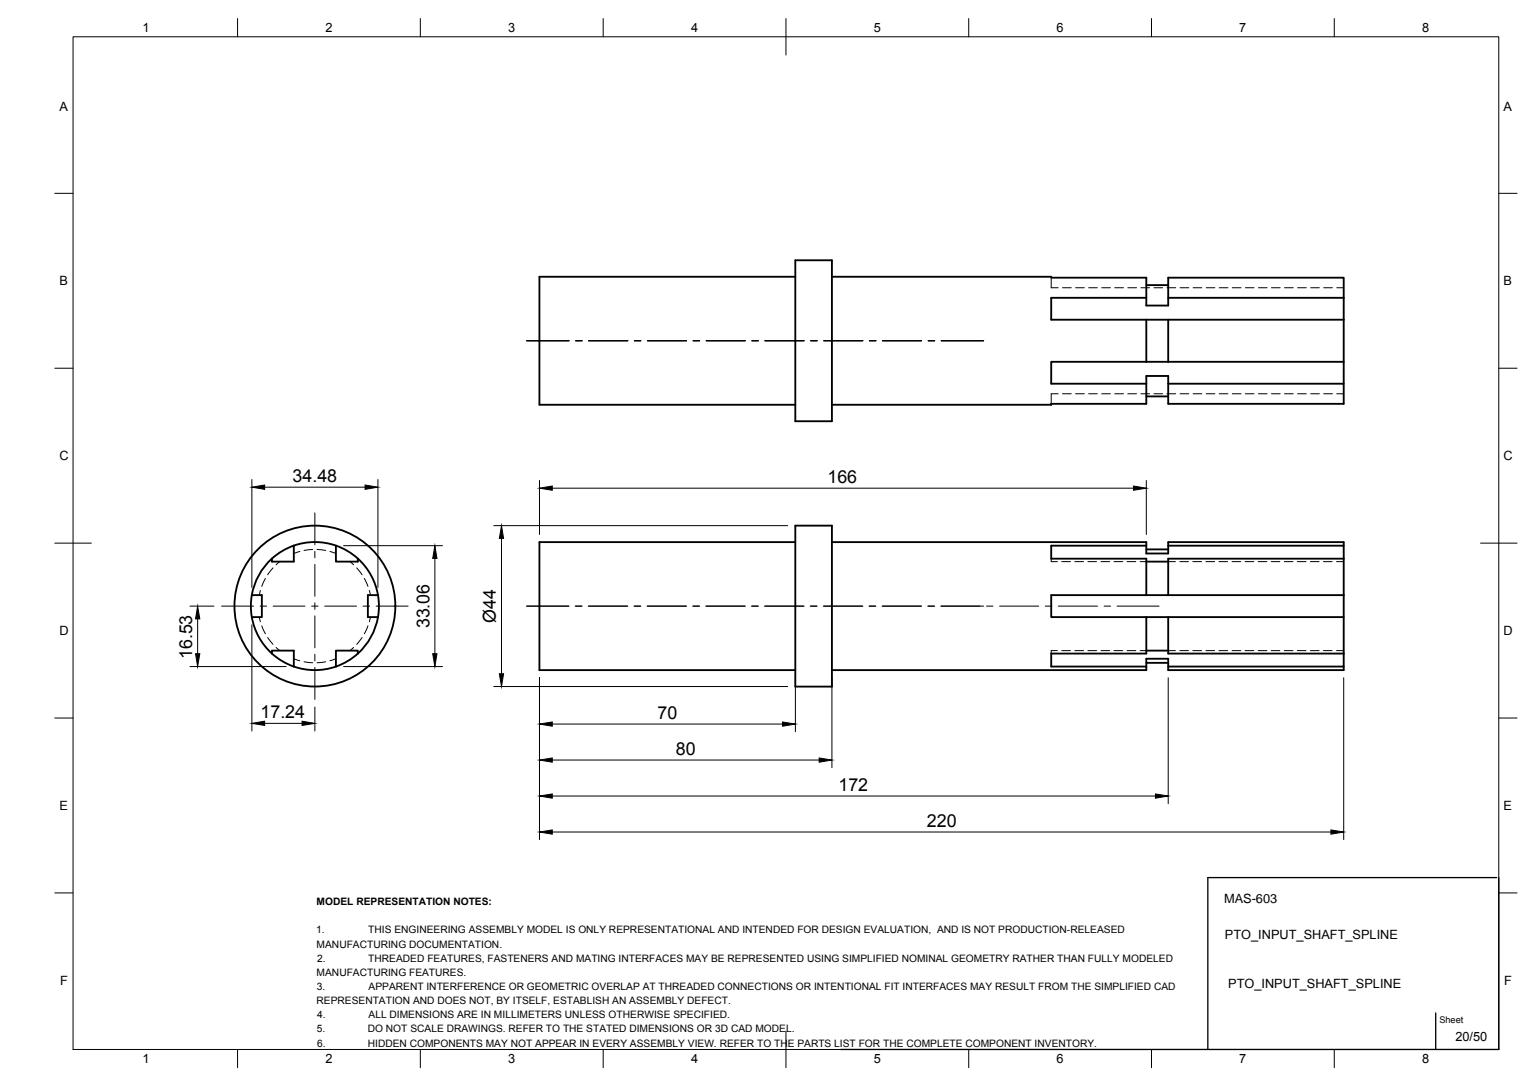
ISO-10303-21;
HEADER;
FILE_DESCRIPTION((''),'2;1');
FILE_NAME('PTO_INPUT_SHAFT_SPLINE.step','2026-10-01T22:06:14-07:00',(''),(''),'','','');
FILE_SCHEMA (('AUTOMOTIVE_DESIGN { 1 0 10303 214 3 1 1 }'));
ENDSEC;
DATA;
#10=MECHANICAL_DESIGN_GEOMETRIC_PRESENTATION_REPRESENTATION('',(#992),#50440);
#902=SHAPE_REPRESENTATION_RELATIONSHIP('SRR','None',#50634,#947) ;
#947=ADVANCED_BREP_SHAPE_REPRESENTATION('',(#1047),#50403) ;
#992=STYLED_ITEM('',(#50883),#1047) ;
#1047=MANIFOLD_SOLID_BREP('PTO_INPUT_SHAFT_SPLINE',#28659) ;
#1295=FACE_BOUND('',#4895,.T.) ;
#1296=FACE_BOUND('',#4898,.T.) ;
#1988=PLANE('',#30408) ;
#1989=PLANE('',#30411) ;
#1990=PLANE('',#30414) ;
#1991=PLANE('',#30417) ;
#1992=PLANE('',#30420) ;
#1993=PLANE('',#30423) ;
#1994=PLANE('',#30438) ;
#1995=PLANE('',#30440) ;
#1996=PLANE('',#30443) ;
#1997=PLANE('',#30445) ;
#1998=PLANE('',#30447) ;
#1999=PLANE('',#30449) ;
#2000=PLANE('',#30451) ;
#2001=PLANE('',#30452) ;
#2002=PLANE('',#30453) ;
#2003=PLANE('',#30454) ;
#2004=PLANE('',#30455) ;
#2005=PLANE('',#30456) ;
#2006=PLANE('',#30457) ;
#2007=PLANE('',#30458) ;
#2008=PLANE('',#30459) ;
#2009=PLANE('',#30460) ;
#2010=PLANE('',#30461) ;
#2011=PLANE('',#30462) ;
#2012=PLANE('',#30475) ;
#2013=PLANE('',#30477) ;
#2014=PLANE('',#30478) ;
#2015=PLANE('',#30479) ;
#2016=PLANE('',#30480) ;
#2017=PLANE('',#30481) ;
#2018=PLANE('',#30483) ;
#2019=PLANE('',#30485) ;
#2020=PLANE('',#30491) ;
#2021=PLANE('',#30492) ;
#2022=PLANE('',#30493) ;
#2023=PLANE('',#30494) ;
#2024=PLANE('',#30495) ;
#2025=PLANE('',#30496) ;
#2026=PLANE('',#30497) ;
#2027=PLANE('',#30498) ;
#2028=PLANE('',#30499) ;
#2029=PLANE('',#30503) ;
#2030=PLANE('',#30504) ;
#2031=PLANE('',#30508) ;
#3101=FACE_OUTER_BOUND('',#4838,.T.) ;
#3102=FACE_OUTER_BOUND('',#4839,.T.) ;
#3103=FACE_OUTER_BOUND('',#4840,.T.) ;
#3104=FACE_OUTER_BOUND('',#4841,.T.) ;
#3105=FACE_OUTER_BOUND('',#4842,.T.) ;
#3106=FACE_OUTER_BOUND('',#4843,.T.) ;
#3107=FACE_OUTER_BOUND('',#4844,.T.) ;
#3108=FACE_OUTER_BOUND('',#4845,.T.) ;
#3109=FACE_OUTER_BOUND('',#4846,.T.) ;
#3110=FACE_OUTER_BOUND('',#4847,.T.) ;
#3111=FACE_OUTER_BOUND('',#4848,.T.) ;
#3112=FACE_OUTER_BOUND('',#4849,.T.) ;
#3113=FACE_OUTER_BOUND('',#4850,.T.) ;
#3114=FACE_OUTER_BOUND('',#4851,.T.) ;
#3115=FACE_OUTER_BOUND('',#4852,.T.) ;
#3116=FACE_OUTER_BOUND('',#4853,.T.) ;
#3117=FACE_OUTER_BOUND('',#4854,.T.) ;
#3118=FACE_OUTER_BOUND('',#4855,.T.) ;
#3119=FACE_OUTER_BOUND('',#4856,.T.) ;
#3120=FACE_OUTER_BOUND('',#4857,.T.) ;
#3121=FACE_OUTER_BOUND('',#4858,.T.) ;
#3122=FACE_OUTER_BOUND('',#4859,.T.) ;
#3123=FACE_OUTER_BOUND('',#4860,.T.) ;
#3124=FACE_OUTER_BOUND('',#4861,.T.) ;
#3125=FACE_OUTER_BOUND('',#4862,.T.) ;
#3126=FACE_OUTER_BOUND('',#4863,.T.) ;
#3127=FACE_OUTER_BOUND('',#4864,.T.) ;
#3128=FACE_OUTER_BOUND('',#4865,.T.) ;
#3129=FACE_OUTER_BOUND('',#4866,.T.) ;
#3130=FACE_OUTER_BOUND('',#4867,.T.) ;
#3131=FACE_OUTER_BOUND('',#4868,.T.) ;
#3132=FACE_OUTER_BOUND('',#4869,.T.) ;
#3133=FACE_OUTER_BOUND('',#4870,.T.) ;
#3134=FACE_OUTER_BOUND('',#4871,.T.) ;
#3135=FACE_OUTER_BOUND('',#4872,.T.) ;
#3136=FACE_OUTER_BOUND('',#4873,.T.) ;
#3137=FACE_OUTER_BOUND('',#4874,.T.) ;
#3138=FACE_OUTER_BOUND('',#4875,.T.) ;
#3139=FACE_OUTER_BOUND('',#4876,.T.) ;
#3140=FACE_OUTER_BOUND('',#4877,.T.) ;
#3141=FACE_OUTER_BOUND('',#4878,.T.) ;
#3142=FACE_OUTER_BOUND('',#4879,.T.) ;
#3143=FACE_OUTER_BOUND('',#4880,.T.) ;
#3144=FACE_OUTER_BOUND('',#4881,.T.) ;
#3145=FACE_OUTER_BOUND('',#4882,.T.) ;
#3146=FACE_OUTER_BOUND('',#4883,.T.) ;
#3147=FACE_OUTER_BOUND('',#4884,.T.) ;
#3148=FACE_OUTER_BOUND('',#4885,.T.) ;
#3149=FACE_OUTER_BOUND('',#4886,.T.) ;
#3150=FACE_OUTER_BOUND('',#4887,.T.) ;
#3151=FACE_OUTER_BOUND('',#4888,.T.) ;
#3152=FACE_OUTER_BOUND('',#4889,.T.) ;
#3153=FACE_OUTER_BOUND('',#4890,.T.) ;
#3154=FACE_OUTER_BOUND('',#4891,.T.) ;
#3155=FACE_OUTER_BOUND('',#4892,.T.) ;
#3156=FACE_OUTER_BOUND('',#4893,.T.) ;
#3157=FACE_OUTER_BOUND('',#4894,.T.) ;
#3158=FACE_OUTER_BOUND('',#4896,.T.) ;
#3159=FACE_OUTER_BOUND('',#4897,.T.) ;
#4838=EDGE_LOOP('',(#22531,#22532,#22533,#22534,#22535)) ;
#4839=EDGE_LOOP('',(#22536,#22537,#22538,#22539,#22540)) ;
#4840=EDGE_LOOP('',(#22541,#22542,#22543,#22544)) ;
#4841=EDGE_LOOP('',(#22545,#22546,#22547,#22548,#22549)) ;
#4842=EDGE_LOOP('',(#22550,#22551,#22552,#22553,#22554)) ;
#4843=EDGE_LOOP('',(#22555,#22556,#22557,#22558)) ;
#4844=EDGE_LOOP('',(#22559,#22560,#22561,#22562)) ;
#4845=EDGE_LOOP('',(#22563,#22564,#22565,#22566)) ;
#4846=EDGE_LOOP('',(#22567,#22568,#22569,#22570)) ;
#4847=EDGE_LOOP('',(#22571,#22572,#22573,#22574)) ;
#4848=EDGE_LOOP('',(#22575,#22576,#22577,#22578)) ;
#4849=EDGE_LOOP('',(#22579,#22580,#22581,#22582)) ;
#4850=EDGE_LOOP('',(#22583,#22584,#22585,#22586,#22587)) ;
#4851=EDGE_LOOP('',(#22588,#22589,#22590,#22591,#22592)) ;
#4852=EDGE_LOOP('',(#22593,#22594,#22595,#22596,#22597)) ;
#4853=EDGE_LOOP('',(#22598,#22599,#22600,#22601,#22602)) ;
#4854=EDGE_LOOP('',(#22603,#22604,#22605,#22606,#22607)) ;
#4855=EDGE_LOOP('',(#22608,#22609,#22610,#22611)) ;
#4856=EDGE_LOOP('',(#22612,#22613,#22614,#22615,#22616,#22617,#22618,#22619)) ;
#4857=EDGE_LOOP('',(#22620,#22621,#22622,#22623,#22624,#22625,#22626,#22627)) ;
#4858=EDGE_LOOP('',(#22628,#22629,#22630,#22631)) ;
#4859=EDGE_LOOP('',(#22632,#22633,#22634,#22635,#22636,#22637,#22638,#22639)) ;
#4860=EDGE_LOOP('',(#22640,#22641,#22642,#22643)) ;
#4861=EDGE_LOOP('',(#22644,#22645,#22646,#22647)) ;
#4862=EDGE_LOOP('',(#22648,#22649,#22650,#22651,#22652,#22653,#22654,#22655)) ;
#4863=EDGE_LOOP('',(#22656,#22657,#22658,#22659)) ;
#4864=EDGE_LOOP('',(#22660,#22661,#22662,#22663,#22664,#22665,#22666,#22667)) ;
#4865=EDGE_LOOP('',(#22668,#22669,#22670,#22671)) ;
#4866=EDGE_LOOP('',(#22672,#22673,#22674,#22675)) ;
#4867=EDGE_LOOP('',(#22676,#22677,#22678,#22679,#22680,#22681,#22682,#22683)) ;
#4868=EDGE_LOOP('',(#22684,#22685,#22686,#22687)) ;
#4869=EDGE_LOOP('',(#22688,#22689,#22690,#22691)) ;
#4870=EDGE_LOOP('',(#22692,#22693,#22694,#22695)) ;
#4871=EDGE_LOOP('',(#22696,#22697,#22698,#22699)) ;
#4872=EDGE_LOOP('',(#22700,#22701,#22702,#22703)) ;
#4873=EDGE_LOOP('',(#22704,#22705,#22706,#22707)) ;
#4874=EDGE_LOOP('',(#22708,#22709,#22710,#22711)) ;
#4875=EDGE_LOOP('',(#22712,#22713,#22714,#22715,#22716,#22717,#22718,#22719,
#22720,#22721,#22722,#22723,#22724,#22725,#22726,#22727,#22728,#22729,#22730,
#22731,#22732,#22733,#22734,#22735)) ;
#4876=EDGE_LOOP('',(#22736,#22737,#22738,#22739,#22740,#22741,#22742,#22743)) ;
#4877=EDGE_LOOP('',(#22744,#22745,#22746,#22747)) ;
#4878=EDGE_LOOP('',(#22748,#22749,#22750,#22751,#22752,#22753,#22754,#22755)) ;
#4879=EDGE_LOOP('',(#22756,#22757,#22758,#22759)) ;
#4880=EDGE_LOOP('',(#22760,#22761,#22762,#22763)) ;
#4881=EDGE_LOOP('',(#22764,#22765,#22766,#22767)) ;
#4882=EDGE_LOOP('',(#22768,#22769,#22770,#22771,#22772,#22773,#22774,#22775,
#22776,#22777,#22778,#22779,#22780,#22781,#22782,#22783,#22784,#22785,#22786,
#22787,#22788,#22789,#22790,#22791,#22792,#22793,#22794,#22795)) ;
#4883=EDGE_LOOP('',(#22796,#22797,#22798,#22799)) ;
#4884=EDGE_LOOP('',(#22800,#22801,#22802,#22803,#22804,#22805,#22806,#22807)) ;
#4885=EDGE_LOOP('',(#22808,#22809,#22810,#22811,#22812,#22813,#22814,#22815)) ;
#4886=EDGE_LOOP('',(#22816,#22817,#22818,#22819)) ;
#4887=EDGE_LOOP('',(#22820,#22821,#22822,#22823,#22824,#22825,#22826,#22827)) ;
#4888=EDGE_LOOP('',(#22828,#22829,#22830,#22831)) ;
#4889=EDGE_LOOP('',(#22832,#22833,#22834,#22835,#22836,#22837,#22838,#22839)) ;
#4890=EDGE_LOOP('',(#22840,#22841,#22842,#22843)) ;
#4891=EDGE_LOOP('',(#22844,#22845,#22846,#22847)) ;
#4892=EDGE_LOOP('',(#22848,#22849,#22850,#22851)) ;
#4893=EDGE_LOOP('',(#22852)) ;
#4894=EDGE_LOOP('',(#22853)) ;
#4895=EDGE_LOOP('',(#22854)) ;
#4896=EDGE_LOOP('',(#22855,#22856,#22857,#22858)) ;
#4897=EDGE_LOOP('',(#22859)) ;
#4898=EDGE_LOOP('',(#22860)) ;
#7284=LINE('',#45461,#9756) ;
#7285=LINE('',#45465,#9757) ;
#7286=LINE('',#45467,#9758) ;
#7287=LINE('',#45472,#9759) ;
#7288=LINE('',#45476,#9760) ;
#7289=LINE('',#45478,#9761) ;
#7290=LINE('',#45483,#9762) ;
#7291=LINE('',#45487,#9763) ;
#7292=LINE('',#45492,#9764) ;
#7293=LINE('',#45496,#9765) ;
#7294=LINE('',#45499,#9766) ;
#7295=LINE('',#45503,#9767) ;
#7296=LINE('',#45507,#9768) ;
#7297=LINE('',#45509,#9769) ;
#7298=LINE('',#45514,#9770) ;
#7299=LINE('',#45518,#9771) ;
#7300=LINE('',#45522,#9772) ;
#7301=LINE('',#45525,#9773) ;
#7302=LINE('',#45528,#9774) ;
#7303=LINE('',#45531,#9775) ;
#7304=LINE('',#45534,#9776) ;
#7305=LINE('',#45536,#9777) ;
#7306=LINE('',#45540,#9778) ;
#7307=LINE('',#45543,#9779) ;
#7308=LINE('',#45546,#9780) ;
#7309=LINE('',#45549,#9781) ;
#7310=LINE('',#45552,#9782) ;
#7311=LINE('',#45555,#9783) ;
#7312=LINE('',#45558,#9784) ;
#7313=LINE('',#45560,#9785) ;
#7314=LINE('',#45562,#9786) ;
#7315=LINE('',#45566,#9787) ;
#7316=LINE('',#45571,#9788) ;
#7317=LINE('',#45574,#9789) ;
#7318=LINE('',#45576,#9790) ;
#7319=LINE('',#45579,#9791) ;
#7320=LINE('',#45582,#9792) ;
#7321=LINE('',#45586,#9793) ;
#7322=LINE('',#45587,#9794) ;
#7323=LINE('',#45590,#9795) ;
#7324=LINE('',#45594,#9796) ;
#7325=LINE('',#45595,#9797) ;
#7326=LINE('',#45598,#9798) ;
#7327=LINE('',#45601,#9799) ;
#7328=LINE('',#45604,#9800) ;
#7329=LINE('',#45606,#9801) ;
#7330=LINE('',#45608,#9802) ;
#7331=LINE('',#45610,#9803) ;
#7332=LINE('',#45611,#9804) ;
#7333=LINE('',#45614,#9805) ;
#7334=LINE('',#45616,#9806) ;
#7335=LINE('',#45618,#9807) ;
#7336=LINE('',#45620,#9808) ;
#7337=LINE('',#45621,#9809) ;
#7338=LINE('',#45624,#9810) ;
#7339=LINE('',#45626,#9811) ;
#7340=LINE('',#45627,#9812) ;
#7341=LINE('',#45630,#9813) ;
#7342=LINE('',#45631,#9814) ;
#7343=LINE('',#45633,#9815) ;
#7344=LINE('',#45634,#9816) ;
#7345=LINE('',#45637,#9817) ;
#7346=LINE('',#45638,#9818) ;
#7347=LINE('',#45641,#9819) ;
#7348=LINE('',#45642,#9820) ;
#7349=LINE('',#45645,#9821) ;
#7350=LINE('',#45647,#9822) ;
#7351=LINE('',#45649,#9823) ;
#7352=LINE('',#45651,#9824) ;
#7353=LINE('',#45652,#9825) ;
#7354=LINE('',#45655,#9826) ;
#7355=LINE('',#45657,#9827) ;
#7356=LINE('',#45658,#9828) ;
#7357=LINE('',#45661,#9829) ;
#7358=LINE('',#45663,#9830) ;
#7359=LINE('',#45665,#9831) ;
#7360=LINE('',#45667,#9832) ;
#7361=LINE('',#45668,#9833) ;
#7362=LINE('',#45671,#9834) ;
#7363=LINE('',#45673,#9835) ;
#7364=LINE('',#45674,#9836) ;
#7365=LINE('',#45677,#9837) ;
#7366=LINE('',#45679,#9838) ;
#7367=LINE('',#45680,#9839) ;
#7368=LINE('',#45683,#9840) ;
#7369=LINE('',#45685,#9841) ;
#7370=LINE('',#45687,#9842) ;
#7371=LINE('',#45689,#9843) ;
#7372=LINE('',#45690,#9844) ;
#7373=LINE('',#45694,#9845) ;
#7374=LINE('',#45700,#9846) ;
#7375=LINE('',#45704,#9847) ;
#7376=LINE('',#45709,#9848) ;
#7377=LINE('',#45715,#9849) ;
#7378=LINE('',#45717,#9850) ;
#7379=LINE('',#45718,#9851) ;
#7380=LINE('',#45719,#9852) ;
#7381=LINE('',#45721,#9853) ;
#7382=LINE('',#45722,#9854) ;
#7383=LINE('',#45723,#9855) ;
#7384=LINE('',#45725,#9856) ;
#7385=LINE('',#45726,#9857) ;
#7386=LINE('',#45729,#9858) ;
#7387=LINE('',#45731,#9859) ;
#7388=LINE('',#45732,#9860) ;
#7389=LINE('',#45734,#9861) ;
#7390=LINE('',#45736,#9862) ;
#7391=LINE('',#45741,#9863) ;
#7392=LINE('',#45746,#9864) ;
#7393=LINE('',#45748,#9865) ;
#7394=LINE('',#45751,#9866) ;
#7395=LINE('',#45753,#9867) ;
#7396=LINE('',#45758,#9868) ;
#7397=LINE('',#45759,#9869) ;
#7398=LINE('',#45762,#9870) ;
#7399=LINE('',#45763,#9871) ;
#7400=LINE('',#45765,#9872) ;
#7401=LINE('',#45768,#9873) ;
#7402=LINE('',#45772,#9874) ;
#7403=LINE('',#45773,#9875) ;
#7404=LINE('',#45775,#9876) ;
#7405=LINE('',#45781,#9877) ;
#7406=LINE('',#45790,#9878) ;
#9756=VECTOR('',#36327,1.) ;
#9757=VECTOR('',#36330,1.) ;
#9758=VECTOR('',#36331,1.) ;
#9759=VECTOR('',#36336,1.) ;
#9760=VECTOR('',#36339,1.) ;
#9761=VECTOR('',#36340,1.) ;
#9762=VECTOR('',#36345,1.) ;
#9763=VECTOR('',#36348,1.) ;
#9764=VECTOR('',#36353,1.) ;
#9765=VECTOR('',#36356,1.) ;
#9766=VECTOR('',#36359,1.) ;
#9767=VECTOR('',#36362,1.) ;
#9768=VECTOR('',#36365,1.) ;
#9769=VECTOR('',#36366,1.) ;
#9770=VECTOR('',#36371,1.) ;
#9771=VECTOR('',#36374,1.) ;
#9772=VECTOR('',#36379,1.) ;
#9773=VECTOR('',#36382,1.) ;
#9774=VECTOR('',#36385,1.) ;
#9775=VECTOR('',#36388,1.) ;
#9776=VECTOR('',#36391,1.) ;
#9777=VECTOR('',#36392,1.) ;
#9778=VECTOR('',#36397,1.) ;
#9779=VECTOR('',#36400,1.) ;
#9780=VECTOR('',#36403,1.) ;
#9781=VECTOR('',#36406,1.) ;
#9782=VECTOR('',#36409,1.) ;
#9783=VECTOR('',#36412,1.) ;
#9784=VECTOR('',#36415,1.) ;
#9785=VECTOR('',#36416,1.) ;
#9786=VECTOR('',#36417,1.) ;
#9787=VECTOR('',#36422,1.) ;
#9788=VECTOR('',#36427,1.) ;
#9789=VECTOR('',#36430,1.) ;
#9790=VECTOR('',#36431,1.) ;
#9791=VECTOR('',#36434,1.) ;
#9792=VECTOR('',#36437,1.) ;
#9793=VECTOR('',#36440,1.) ;
#9794=VECTOR('',#36441,1.) ;
#9795=VECTOR('',#36444,1.) ;
#9796=VECTOR('',#36447,1.) ;
#9797=VECTOR('',#36448,1.) ;
#9798=VECTOR('',#36451,1.) ;
#9799=VECTOR('',#36454,1.) ;
#9800=VECTOR('',#36457,1.) ;
#9801=VECTOR('',#36458,1.) ;
#9802=VECTOR('',#36459,1.) ;
#9803=VECTOR('',#36460,1.) ;
#9804=VECTOR('',#36461,1.) ;
#9805=VECTOR('',#36464,1.) ;
#9806=VECTOR('',#36465,1.) ;
#9807=VECTOR('',#36466,1.) ;
#9808=VECTOR('',#36467,1.) ;
#9809=VECTOR('',#36468,1.) ;
#9810=VECTOR('',#36471,1.) ;
#9811=VECTOR('',#36472,1.) ;
#9812=VECTOR('',#36473,1.) ;
#9813=VECTOR('',#36476,1.) ;
#9814=VECTOR('',#36477,1.) ;
#9815=VECTOR('',#36478,1.) ;
#9816=VECTOR('',#36479,1.) ;
#9817=VECTOR('',#36482,1.) ;
#9818=VECTOR('',#36483,1.) ;
#9819=VECTOR('',#36486,1.) ;
#9820=VECTOR('',#36487,1.) ;
#9821=VECTOR('',#36490,1.) ;
#9822=VECTOR('',#36491,1.) ;
#9823=VECTOR('',#36492,1.) ;
#9824=VECTOR('',#36493,1.) ;
#9825=VECTOR('',#36494,1.) ;
#9826=VECTOR('',#36497,1.) ;
#9827=VECTOR('',#36498,1.) ;
#9828=VECTOR('',#36499,1.) ;
#9829=VECTOR('',#36502,1.) ;
#9830=VECTOR('',#36503,1.) ;
#9831=VECTOR('',#36504,1.) ;
#9832=VECTOR('',#36505,1.) ;
#9833=VECTOR('',#36506,1.) ;
#9834=VECTOR('',#36509,1.) ;
#9835=VECTOR('',#36510,1.) ;
#9836=VECTOR('',#36511,1.) ;
#9837=VECTOR('',#36514,1.) ;
#9838=VECTOR('',#36515,1.) ;
#9839=VECTOR('',#36516,1.) ;
#9840=VECTOR('',#36519,1.) ;
#9841=VECTOR('',#36520,1.) ;
#9842=VECTOR('',#36521,1.) ;
#9843=VECTOR('',#36522,1.) ;
#9844=VECTOR('',#36523,1.) ;
#9845=VECTOR('',#36528,1.) ;
#9846=VECTOR('',#36537,1.) ;
#9847=VECTOR('',#36542,1.) ;
#9848=VECTOR('',#36549,1.) ;
#9849=VECTOR('',#36558,1.) ;
#9850=VECTOR('',#36559,1.) ;
#9851=VECTOR('',#36560,1.) ;
#9852=VECTOR('',#36561,1.) ;
#9853=VECTOR('',#36562,1.) ;
#9854=VECTOR('',#36563,1.) ;
#9855=VECTOR('',#36564,1.) ;
#9856=VECTOR('',#36565,1.) ;
#9857=VECTOR('',#36566,1.) ;
#9858=VECTOR('',#36569,1.) ;
#9859=VECTOR('',#36570,1.) ;
#9860=VECTOR('',#36571,1.) ;
#9861=VECTOR('',#36574,1.) ;
#9862=VECTOR('',#36577,1.) ;
#9863=VECTOR('',#36586,1.) ;
#9864=VECTOR('',#36593,1.75) ;
#9865=VECTOR('',#36594,1.) ;
#9866=VECTOR('',#36597,1.) ;
#9867=VECTOR('',#36598,1.) ;
#9868=VECTOR('',#36605,1.) ;
#9869=VECTOR('',#36606,1.) ;
#9870=VECTOR('',#36609,1.) ;
#9871=VECTOR('',#36610,1.) ;
#9872=VECTOR('',#36613,1.) ;
#9873=VECTOR('',#36618,1.) ;
#9874=VECTOR('',#36623,1.) ;
#9875=VECTOR('',#36624,1.) ;
#9876=VECTOR('',#36627,1.) ;
#9877=VECTOR('',#36634,1.75) ;
#9878=VECTOR('',#36647,2.2) ;
#11051=CIRCLE('',#30409,1.75) ;
#11052=CIRCLE('',#30410,1.55) ;
#11053=CIRCLE('',#30412,1.55) ;
#11054=CIRCLE('',#30413,1.75) ;
#11055=CIRCLE('',#30415,1.55) ;
#11056=CIRCLE('',#30416,1.75) ;
#11057=CIRCLE('',#30418,1.55) ;
#11058=CIRCLE('',#30419,1.75) ;
#11059=CIRCLE('',#30421,1.55) ;
#11060=CIRCLE('',#30422,1.75) ;
#11061=CIRCLE('',#30424,1.55) ;
#11062=CIRCLE('',#30425,1.75) ;
#11063=CIRCLE('',#30427,1.55) ;
#11064=CIRCLE('',#30429,1.55) ;
#11065=CIRCLE('',#30431,1.55) ;
#11066=CIRCLE('',#30433,1.55) ;
#11067=CIRCLE('',#30435,1.55) ;
#11068=CIRCLE('',#30437,1.55) ;
#11069=CIRCLE('',#30439,1.75) ;
#11070=CIRCLE('',#30441,1.75) ;
#11071=CIRCLE('',#30442,1.75) ;
#11072=CIRCLE('',#30444,1.75) ;
#11073=CIRCLE('',#30446,1.75) ;
#11074=CIRCLE('',#30448,1.75) ;
#11075=CIRCLE('',#30450,1.75) ;
#11076=CIRCLE('',#30464,1.75) ;
#11077=CIRCLE('',#30466,1.75) ;
#11078=CIRCLE('',#30468,1.75) ;
#11079=CIRCLE('',#30470,1.75) ;
#11080=CIRCLE('',#30472,1.75) ;
#11081=CIRCLE('',#30474,1.75) ;
#11082=CIRCLE('',#30476,1.75) ;
#11083=CIRCLE('',#30482,1.75) ;
#11084=CIRCLE('',#30484,1.75) ;
#11085=CIRCLE('',#30487,1.75) ;
#11086=CIRCLE('',#30488,1.75) ;
#11087=CIRCLE('',#30489,1.75) ;
#11088=CIRCLE('',#30490,1.75) ;
#11089=CIRCLE('',#30501,1.75) ;
#11090=CIRCLE('',#30502,1.75) ;
#11091=CIRCLE('',#30505,2.2) ;
#11092=CIRCLE('',#30507,2.2) ;
#13161=VERTEX_POINT('',#45459) ;
#13162=VERTEX_POINT('',#45460) ;
#13163=VERTEX_POINT('',#45462) ;
#13164=VERTEX_POINT('',#45464) ;
#13165=VERTEX_POINT('',#45466) ;
#13166=VERTEX_POINT('',#45470) ;
#13167=VERTEX_POINT('',#45471) ;
#13168=VERTEX_POINT('',#45473) ;
#13169=VERTEX_POINT('',#45475) ;
#13170=VERTEX_POINT('',#45477) ;
#13171=VERTEX_POINT('',#45481) ;
#13172=VERTEX_POINT('',#45482) ;
#13173=VERTEX_POINT('',#45484) ;
#13174=VERTEX_POINT('',#45486) ;
#13175=VERTEX_POINT('',#45490) ;
#13176=VERTEX_POINT('',#45491) ;
#13177=VERTEX_POINT('',#45493) ;
#13178=VERTEX_POINT('',#45495) ;
#13179=VERTEX_POINT('',#45497) ;
#13180=VERTEX_POINT('',#45501) ;
#13181=VERTEX_POINT('',#45502) ;
#13182=VERTEX_POINT('',#45504) ;
#13183=VERTEX_POINT('',#45506) ;
#13184=VERTEX_POINT('',#45508) ;
#13185=VERTEX_POINT('',#45512) ;
#13186=VERTEX_POINT('',#45513) ;
#13187=VERTEX_POINT('',#45515) ;
#13188=VERTEX_POINT('',#45517) ;
#13189=VERTEX_POINT('',#45521) ;
#13190=VERTEX_POINT('',#45523) ;
#13191=VERTEX_POINT('',#45527) ;
#13192=VERTEX_POINT('',#45529) ;
#13193=VERTEX_POINT('',#45533) ;
#13194=VERTEX_POINT('',#45535) ;
#13195=VERTEX_POINT('',#45539) ;
#13196=VERTEX_POINT('',#45541) ;
#13197=VERTEX_POINT('',#45545) ;
#13198=VERTEX_POINT('',#45547) ;
#13199=VERTEX_POINT('',#45551) ;
#13200=VERTEX_POINT('',#45553) ;
#13201=VERTEX_POINT('',#45557) ;
#13202=VERTEX_POINT('',#45559) ;
#13203=VERTEX_POINT('',#45561) ;
#13204=VERTEX_POINT('',#45565) ;
#13205=VERTEX_POINT('',#45567) ;
#13206=VERTEX_POINT('',#45569) ;
#13207=VERTEX_POINT('',#45573) ;
#13208=VERTEX_POINT('',#45575) ;
#13209=VERTEX_POINT('',#45577) ;
#13210=VERTEX_POINT('',#45581) ;
#13211=VERTEX_POINT('',#45583) ;
#13212=VERTEX_POINT('',#45585) ;
#13213=VERTEX_POINT('',#45589) ;
#13214=VERTEX_POINT('',#45591) ;
#13215=VERTEX_POINT('',#45593) ;
#13216=VERTEX_POINT('',#45597) ;
#13217=VERTEX_POINT('',#45599) ;
#13218=VERTEX_POINT('',#45603) ;
#13219=VERTEX_POINT('',#45605) ;
#13220=VERTEX_POINT('',#45607) ;
#13221=VERTEX_POINT('',#45609) ;
#13222=VERTEX_POINT('',#45613) ;
#13223=VERTEX_POINT('',#45615) ;
#13224=VERTEX_POINT('',#45617) ;
#13225=VERTEX_POINT('',#45619) ;
#13226=VERTEX_POINT('',#45623) ;
#13227=VERTEX_POINT('',#45625) ;
#13228=VERTEX_POINT('',#45629) ;
#13229=VERTEX_POINT('',#45632) ;
#13230=VERTEX_POINT('',#45636) ;
#13231=VERTEX_POINT('',#45640) ;
#13232=VERTEX_POINT('',#45644) ;
#13233=VERTEX_POINT('',#45646) ;
#13234=VERTEX_POINT('',#45648) ;
#13235=VERTEX_POINT('',#45650) ;
#13236=VERTEX_POINT('',#45654) ;
#13237=VERTEX_POINT('',#45656) ;
#13238=VERTEX_POINT('',#45660) ;
#13239=VERTEX_POINT('',#45662) ;
#13240=VERTEX_POINT('',#45664) ;
#13241=VERTEX_POINT('',#45666) ;
#13242=VERTEX_POINT('',#45670) ;
#13243=VERTEX_POINT('',#45672) ;
#13244=VERTEX_POINT('',#45676) ;
#13245=VERTEX_POINT('',#45678) ;
#13246=VERTEX_POINT('',#45682) ;
#13247=VERTEX_POINT('',#45684) ;
#13248=VERTEX_POINT('',#45686) ;
#13249=VERTEX_POINT('',#45688) ;
#13250=VERTEX_POINT('',#45692) ;
#13251=VERTEX_POINT('',#45698) ;
#13252=VERTEX_POINT('',#45702) ;
#13253=VERTEX_POINT('',#45708) ;
#13254=VERTEX_POINT('',#45714) ;
#13255=VERTEX_POINT('',#45716) ;
#13256=VERTEX_POINT('',#45720) ;
#13257=VERTEX_POINT('',#45724) ;
#13258=VERTEX_POINT('',#45728) ;
#13259=VERTEX_POINT('',#45730) ;
#13260=VERTEX_POINT('',#45744) ;
#13261=VERTEX_POINT('',#45747) ;
#13262=VERTEX_POINT('',#45749) ;
#13263=VERTEX_POINT('',#45752) ;
#13264=VERTEX_POINT('',#45757) ;
#13265=VERTEX_POINT('',#45761) ;
#13266=VERTEX_POINT('',#45771) ;
#13267=VERTEX_POINT('',#45778) ;
#13268=VERTEX_POINT('',#45780) ;
#13269=VERTEX_POINT('',#45785) ;
#13270=VERTEX_POINT('',#45788) ;
#16531=EDGE_CURVE('',#13161,#13162,#7284,.T.) ;
#16532=EDGE_CURVE('',#13163,#13161,#11051,.T.) ;
#16533=EDGE_CURVE('',#13164,#13163,#7285,.T.) ;
#16534=EDGE_CURVE('',#13165,#13164,#7286,.T.) ;
#16535=EDGE_CURVE('',#13162,#13165,#11052,.T.) ;
#16536=EDGE_CURVE('',#13166,#13167,#7287,.T.) ;
#16537=EDGE_CURVE('',#13168,#13166,#11053,.T.) ;
#16538=EDGE_CURVE('',#13169,#13168,#7288,.T.) ;
#16539=EDGE_CURVE('',#13170,#13169,#7289,.T.) ;
#16540=EDGE_CURVE('',#13167,#13170,#11054,.T.) ;
#16541=EDGE_CURVE('',#13171,#13172,#7290,.T.) ;
#16542=EDGE_CURVE('',#13173,#13171,#11055,.T.) ;
#16543=EDGE_CURVE('',#13174,#13173,#7291,.T.) ;
#16544=EDGE_CURVE('',#13172,#13174,#11056,.T.) ;
#16545=EDGE_CURVE('',#13175,#13176,#7292,.T.) ;
#16546=EDGE_CURVE('',#13177,#13175,#11057,.T.) ;
#16547=EDGE_CURVE('',#13178,#13177,#7293,.T.) ;
#16548=EDGE_CURVE('',#13179,#13178,#11058,.T.) ;
#16549=EDGE_CURVE('',#13176,#13179,#7294,.T.) ;
#16550=EDGE_CURVE('',#13180,#13181,#7295,.T.) ;
#16551=EDGE_CURVE('',#13182,#13180,#11059,.T.) ;
#16552=EDGE_CURVE('',#13183,#13182,#7296,.T.) ;
#16553=EDGE_CURVE('',#13184,#13183,#7297,.T.) ;
#16554=EDGE_CURVE('',#13181,#13184,#11060,.T.) ;
#16555=EDGE_CURVE('',#13185,#13186,#7298,.T.) ;
#16556=EDGE_CURVE('',#13187,#13185,#11061,.T.) ;
#16557=EDGE_CURVE('',#13188,#13187,#7299,.T.) ;
#16558=EDGE_CURVE('',#13186,#13188,#11062,.T.) ;
#16559=EDGE_CURVE('',#13189,#13175,#7300,.T.) ;
#16560=EDGE_CURVE('',#13189,#13190,#11063,.T.) ;
#16561=EDGE_CURVE('',#13177,#13190,#7301,.T.) ;
#16562=EDGE_CURVE('',#13191,#13171,#7302,.T.) ;
#16563=EDGE_CURVE('',#13191,#13192,#11064,.T.) ;
#16564=EDGE_CURVE('',#13173,#13192,#7303,.T.) ;
#16565=EDGE_CURVE('',#13162,#13193,#7304,.T.) ;
#16566=EDGE_CURVE('',#13194,#13165,#7305,.T.) ;
#16567=EDGE_CURVE('',#13194,#13193,#11065,.T.) ;
#16568=EDGE_CURVE('',#13195,#13166,#7306,.T.) ;
#16569=EDGE_CURVE('',#13195,#13196,#11066,.T.) ;
#16570=EDGE_CURVE('',#13168,#13196,#7307,.T.) ;
#16571=EDGE_CURVE('',#13197,#13180,#7308,.T.) ;
#16572=EDGE_CURVE('',#13197,#13198,#11067,.T.) ;
#16573=EDGE_CURVE('',#13182,#13198,#7309,.T.) ;
#16574=EDGE_CURVE('',#13199,#13185,#7310,.T.) ;
#16575=EDGE_CURVE('',#13199,#13200,#11068,.T.) ;
#16576=EDGE_CURVE('',#13187,#13200,#7311,.T.) ;
#16577=EDGE_CURVE('',#13193,#13201,#7312,.T.) ;
#16578=EDGE_CURVE('',#13202,#13194,#7313,.T.) ;
#16579=EDGE_CURVE('',#13203,#13202,#7314,.T.) ;
#16580=EDGE_CURVE('',#13201,#13203,#11069,.T.) ;
#16581=EDGE_CURVE('',#13204,#13191,#7315,.T.) ;
#16582=EDGE_CURVE('',#13205,#13204,#11070,.T.) ;
#16583=EDGE_CURVE('',#13206,#13205,#11071,.T.) ;
#16584=EDGE_CURVE('',#13192,#13206,#7316,.T.) ;
#16585=EDGE_CURVE('',#13207,#13189,#7317,.T.) ;
#16586=EDGE_CURVE('',#13208,#13207,#7318,.T.) ;
#16587=EDGE_CURVE('',#13209,#13208,#11072,.T.) ;
#16588=EDGE_CURVE('',#13190,#13209,#7319,.T.) ;
#16589=EDGE_CURVE('',#13210,#13197,#7320,.T.) ;
#16590=EDGE_CURVE('',#13211,#13210,#11073,.T.) ;
#16591=EDGE_CURVE('',#13212,#13211,#7321,.T.) ;
#16592=EDGE_CURVE('',#13198,#13212,#7322,.T.) ;
#16593=EDGE_CURVE('',#13213,#13195,#7323,.T.) ;
#16594=EDGE_CURVE('',#13214,#13213,#11074,.T.) ;
#16595=EDGE_CURVE('',#13215,#13214,#7324,.T.) ;
#16596=EDGE_CURVE('',#13196,#13215,#7325,.T.) ;
#16597=EDGE_CURVE('',#13216,#13199,#7326,.T.) ;
#16598=EDGE_CURVE('',#13217,#13216,#11075,.T.) ;
#16599=EDGE_CURVE('',#13200,#13217,#7327,.T.) ;
#16600=EDGE_CURVE('',#13218,#13186,#7328,.T.) ;
#16601=EDGE_CURVE('',#13219,#13218,#7329,.T.) ;
#16602=EDGE_CURVE('',#13220,#13219,#7330,.T.) ;
#16603=EDGE_CURVE('',#13221,#13220,#7331,.T.) ;
#16604=EDGE_CURVE('',#13216,#13221,#7332,.T.) ;
#16605=EDGE_CURVE('',#13222,#13167,#7333,.T.) ;
#16606=EDGE_CURVE('',#13223,#13222,#7334,.T.) ;
#16607=EDGE_CURVE('',#13224,#13223,#7335,.T.) ;
#16608=EDGE_CURVE('',#13225,#13224,#7336,.T.) ;
#16609=EDGE_CURVE('',#13213,#13225,#7337,.T.) ;
#16610=EDGE_CURVE('',#13226,#13169,#7338,.T.) ;
#16611=EDGE_CURVE('',#13227,#13226,#7339,.T.) ;
#16612=EDGE_CURVE('',#13170,#13227,#7340,.T.) ;
#16613=EDGE_CURVE('',#13212,#13228,#7341,.T.) ;
#16614=EDGE_CURVE('',#13228,#13220,#7342,.T.) ;
#16615=EDGE_CURVE('',#13229,#13219,#7343,.T.) ;
#16616=EDGE_CURVE('',#13229,#13183,#7344,.T.) ;
#16617=EDGE_CURVE('',#13230,#13211,#7345,.T.) ;
#16618=EDGE_CURVE('',#13228,#13230,#7346,.T.) ;
#16619=EDGE_CURVE('',#13231,#13229,#7347,.T.) ;
#16620=EDGE_CURVE('',#13184,#13231,#7348,.T.) ;
#16621=EDGE_CURVE('',#13232,#13201,#7349,.T.) ;
#16622=EDGE_CURVE('',#13233,#13232,#7350,.T.) ;
#16623=EDGE_CURVE('',#13234,#13233,#7351,.T.) ;
#16624=EDGE_CURVE('',#13235,#13234,#7352,.T.) ;
#16625=EDGE_CURVE('',#13161,#13235,#7353,.T.) ;
#16626=EDGE_CURVE('',#13236,#13202,#7354,.T.) ;
#16627=EDGE_CURVE('',#13237,#13236,#7355,.T.) ;
#16628=EDGE_CURVE('',#13203,#13237,#7356,.T.) ;
#16629=EDGE_CURVE('',#13238,#13209,#7357,.T.) ;
#16630=EDGE_CURVE('',#13239,#13238,#7358,.T.) ;
#16631=EDGE_CURVE('',#13240,#13239,#7359,.T.) ;
#16632=EDGE_CURVE('',#13241,#13240,#7360,.T.) ;
#16633=EDGE_CURVE('',#13178,#13241,#7361,.T.) ;
#16634=EDGE_CURVE('',#13242,#13207,#7362,.T.) ;
#16635=EDGE_CURVE('',#13243,#13242,#7363,.T.) ;
#16636=EDGE_CURVE('',#13208,#13243,#7364,.T.) ;
#16637=EDGE_CURVE('',#13244,#13179,#7365,.T.) ;
#16638=EDGE_CURVE('',#13245,#13244,#7366,.T.) ;
#16639=EDGE_CURVE('',#13176,#13245,#7367,.T.) ;
#16640=EDGE_CURVE('',#13246,#13206,#7368,.T.) ;
#16641=EDGE_CURVE('',#13247,#13246,#7369,.T.) ;
#16642=EDGE_CURVE('',#13248,#13247,#7370,.T.) ;
#16643=EDGE_CURVE('',#13249,#13248,#7371,.T.) ;
#16644=EDGE_CURVE('',#13174,#13249,#7372,.T.) ;
#16645=EDGE_CURVE('',#13250,#13249,#11076,.T.) ;
#16646=EDGE_CURVE('',#13250,#13172,#7373,.T.) ;
#16647=EDGE_CURVE('',#13244,#13241,#11077,.T.) ;
#16648=EDGE_CURVE('',#13251,#13231,#11078,.T.) ;
#16649=EDGE_CURVE('',#13251,#13181,#7374,.T.) ;
#16650=EDGE_CURVE('',#13252,#13235,#11079,.T.) ;
#16651=EDGE_CURVE('',#13252,#13163,#7375,.T.) ;
#16652=EDGE_CURVE('',#13222,#13227,#11080,.T.) ;
#16653=EDGE_CURVE('',#13188,#13253,#7376,.T.) ;
#16654=EDGE_CURVE('',#13218,#13253,#11081,.T.) ;
#16655=EDGE_CURVE('',#13221,#13230,#11082,.T.) ;
#16656=EDGE_CURVE('',#13253,#13254,#7377,.T.) ;
#16657=EDGE_CURVE('',#13254,#13255,#7378,.T.) ;
#16658=EDGE_CURVE('',#13255,#13252,#7379,.T.) ;
#16659=EDGE_CURVE('',#13234,#13223,#7380,.T.) ;
#16660=EDGE_CURVE('',#13226,#13256,#7381,.T.) ;
#16661=EDGE_CURVE('',#13256,#13250,#7382,.T.) ;
#16662=EDGE_CURVE('',#13248,#13245,#7383,.T.) ;
#16663=EDGE_CURVE('',#13240,#13257,#7384,.T.) ;
#16664=EDGE_CURVE('',#13257,#13251,#7385,.T.) ;
#16665=EDGE_CURVE('',#13258,#13217,#7386,.T.) ;
#16666=EDGE_CURVE('',#13259,#13258,#7387,.T.) ;
#16667=EDGE_CURVE('',#13254,#13259,#7388,.T.) ;
#16668=EDGE_CURVE('',#13164,#13255,#7389,.T.) ;
#16669=EDGE_CURVE('',#13259,#13236,#7390,.T.) ;
#16670=EDGE_CURVE('',#13237,#13258,#11083,.T.) ;
#16671=EDGE_CURVE('',#13225,#13232,#11084,.T.) ;
#16672=EDGE_CURVE('',#13224,#13233,#7391,.T.) ;
#16673=EDGE_CURVE('',#13260,#13260,#11085,.T.) ;
#16674=EDGE_CURVE('',#13260,#13205,#7392,.T.) ;
#16675=EDGE_CURVE('',#13204,#13261,#7393,.T.) ;
#16676=EDGE_CURVE('',#13261,#13262,#11086,.T.) ;
#16677=EDGE_CURVE('',#13262,#13214,#7394,.T.) ;
#16678=EDGE_CURVE('',#13210,#13263,#7395,.T.) ;
#16679=EDGE_CURVE('',#13263,#13238,#11087,.T.) ;
#16680=EDGE_CURVE('',#13243,#13246,#11088,.T.) ;
#16681=EDGE_CURVE('',#13264,#13262,#7396,.T.) ;
#16682=EDGE_CURVE('',#13215,#13264,#7397,.T.) ;
#16683=EDGE_CURVE('',#13265,#13256,#7398,.T.) ;
#16684=EDGE_CURVE('',#13261,#13265,#7399,.T.) ;
#16685=EDGE_CURVE('',#13264,#13265,#7400,.T.) ;
#16686=EDGE_CURVE('',#13247,#13242,#7401,.T.) ;
#16687=EDGE_CURVE('',#13266,#13257,#7402,.T.) ;
#16688=EDGE_CURVE('',#13263,#13266,#7403,.T.) ;
#16689=EDGE_CURVE('',#13239,#13266,#7404,.T.) ;
#16690=EDGE_CURVE('',#13267,#13267,#11089,.T.) ;
#16691=EDGE_CURVE('',#13267,#13268,#7405,.T.) ;
#16692=EDGE_CURVE('',#13268,#13268,#11090,.T.) ;
#16693=EDGE_CURVE('',#13269,#13269,#11091,.T.) ;
#16694=EDGE_CURVE('',#13270,#13270,#11092,.T.) ;
#16695=EDGE_CURVE('',#13270,#13269,#7406,.T.) ;
#22531=ORIENTED_EDGE('',*,*,#16531,.F.) ;
#22532=ORIENTED_EDGE('',*,*,#16532,.F.) ;
#22533=ORIENTED_EDGE('',*,*,#16533,.F.) ;
#22534=ORIENTED_EDGE('',*,*,#16534,.F.) ;
#22535=ORIENTED_EDGE('',*,*,#16535,.F.) ;
#22536=ORIENTED_EDGE('',*,*,#16536,.F.) ;
#22537=ORIENTED_EDGE('',*,*,#16537,.F.) ;
#22538=ORIENTED_EDGE('',*,*,#16538,.F.) ;
#22539=ORIENTED_EDGE('',*,*,#16539,.F.) ;
#22540=ORIENTED_EDGE('',*,*,#16540,.F.) ;
#22541=ORIENTED_EDGE('',*,*,#16541,.F.) ;
#22542=ORIENTED_EDGE('',*,*,#16542,.F.) ;
#22543=ORIENTED_EDGE('',*,*,#16543,.F.) ;
#22544=ORIENTED_EDGE('',*,*,#16544,.F.) ;
#22545=ORIENTED_EDGE('',*,*,#16545,.F.) ;
#22546=ORIENTED_EDGE('',*,*,#16546,.F.) ;
#22547=ORIENTED_EDGE('',*,*,#16547,.F.) ;
#22548=ORIENTED_EDGE('',*,*,#16548,.F.) ;
#22549=ORIENTED_EDGE('',*,*,#16549,.F.) ;
#22550=ORIENTED_EDGE('',*,*,#16550,.F.) ;
#22551=ORIENTED_EDGE('',*,*,#16551,.F.) ;
#22552=ORIENTED_EDGE('',*,*,#16552,.F.) ;
#22553=ORIENTED_EDGE('',*,*,#16553,.F.) ;
#22554=ORIENTED_EDGE('',*,*,#16554,.F.) ;
#22555=ORIENTED_EDGE('',*,*,#16555,.F.) ;
#22556=ORIENTED_EDGE('',*,*,#16556,.F.) ;
#22557=ORIENTED_EDGE('',*,*,#16557,.F.) ;
#22558=ORIENTED_EDGE('',*,*,#16558,.F.) ;
#22559=ORIENTED_EDGE('',*,*,#16559,.F.) ;
#22560=ORIENTED_EDGE('',*,*,#16560,.T.) ;
#22561=ORIENTED_EDGE('',*,*,#16561,.F.) ;
#22562=ORIENTED_EDGE('',*,*,#16546,.T.) ;
#22563=ORIENTED_EDGE('',*,*,#16562,.F.) ;
#22564=ORIENTED_EDGE('',*,*,#16563,.T.) ;
#22565=ORIENTED_EDGE('',*,*,#16564,.F.) ;
#22566=ORIENTED_EDGE('',*,*,#16542,.T.) ;
#22567=ORIENTED_EDGE('',*,*,#16565,.F.) ;
#22568=ORIENTED_EDGE('',*,*,#16535,.T.) ;
#22569=ORIENTED_EDGE('',*,*,#16566,.F.) ;
#22570=ORIENTED_EDGE('',*,*,#16567,.T.) ;
#22571=ORIENTED_EDGE('',*,*,#16568,.F.) ;
#22572=ORIENTED_EDGE('',*,*,#16569,.T.) ;
#22573=ORIENTED_EDGE('',*,*,#16570,.F.) ;
#22574=ORIENTED_EDGE('',*,*,#16537,.T.) ;
#22575=ORIENTED_EDGE('',*,*,#16571,.F.) ;
#22576=ORIENTED_EDGE('',*,*,#16572,.T.) ;
#22577=ORIENTED_EDGE('',*,*,#16573,.F.) ;
#22578=ORIENTED_EDGE('',*,*,#16551,.T.) ;
#22579=ORIENTED_EDGE('',*,*,#16574,.F.) ;
#22580=ORIENTED_EDGE('',*,*,#16575,.T.) ;
#22581=ORIENTED_EDGE('',*,*,#16576,.F.) ;
#22582=ORIENTED_EDGE('',*,*,#16556,.T.) ;
#22583=ORIENTED_EDGE('',*,*,#16577,.F.) ;
#22584=ORIENTED_EDGE('',*,*,#16567,.F.) ;
#22585=ORIENTED_EDGE('',*,*,#16578,.F.) ;
#22586=ORIENTED_EDGE('',*,*,#16579,.F.) ;
#22587=ORIENTED_EDGE('',*,*,#16580,.F.) ;
#22588=ORIENTED_EDGE('',*,*,#16581,.F.) ;
#22589=ORIENTED_EDGE('',*,*,#16582,.F.) ;
#22590=ORIENTED_EDGE('',*,*,#16583,.F.) ;
#22591=ORIENTED_EDGE('',*,*,#16584,.F.) ;
#22592=ORIENTED_EDGE('',*,*,#16563,.F.) ;
#22593=ORIENTED_EDGE('',*,*,#16585,.F.) ;
#22594=ORIENTED_EDGE('',*,*,#16586,.F.) ;
#22595=ORIENTED_EDGE('',*,*,#16587,.F.) ;
#22596=ORIENTED_EDGE('',*,*,#16588,.F.) ;
#22597=ORIENTED_EDGE('',*,*,#16560,.F.) ;
#22598=ORIENTED_EDGE('',*,*,#16589,.F.) ;
#22599=ORIENTED_EDGE('',*,*,#16590,.F.) ;
#22600=ORIENTED_EDGE('',*,*,#16591,.F.) ;
#22601=ORIENTED_EDGE('',*,*,#16592,.F.) ;
#22602=ORIENTED_EDGE('',*,*,#16572,.F.) ;
#22603=ORIENTED_EDGE('',*,*,#16593,.F.) ;
#22604=ORIENTED_EDGE('',*,*,#16594,.F.) ;
#22605=ORIENTED_EDGE('',*,*,#16595,.F.) ;
#22606=ORIENTED_EDGE('',*,*,#16596,.F.) ;
#22607=ORIENTED_EDGE('',*,*,#16569,.F.) ;
#22608=ORIENTED_EDGE('',*,*,#16597,.F.) ;
#22609=ORIENTED_EDGE('',*,*,#16598,.F.) ;
#22610=ORIENTED_EDGE('',*,*,#16599,.F.) ;
#22611=ORIENTED_EDGE('',*,*,#16575,.F.) ;
#22612=ORIENTED_EDGE('',*,*,#16597,.T.) ;
#22613=ORIENTED_EDGE('',*,*,#16574,.T.) ;
#22614=ORIENTED_EDGE('',*,*,#16555,.T.) ;
#22615=ORIENTED_EDGE('',*,*,#16600,.F.) ;
#22616=ORIENTED_EDGE('',*,*,#16601,.F.) ;
#22617=ORIENTED_EDGE('',*,*,#16602,.F.) ;
#22618=ORIENTED_EDGE('',*,*,#16603,.F.) ;
#22619=ORIENTED_EDGE('',*,*,#16604,.F.) ;
#22620=ORIENTED_EDGE('',*,*,#16593,.T.) ;
#22621=ORIENTED_EDGE('',*,*,#16568,.T.) ;
#22622=ORIENTED_EDGE('',*,*,#16536,.T.) ;
#22623=ORIENTED_EDGE('',*,*,#16605,.F.) ;
#22624=ORIENTED_EDGE('',*,*,#16606,.F.) ;
#22625=ORIENTED_EDGE('',*,*,#16607,.F.) ;
#22626=ORIENTED_EDGE('',*,*,#16608,.F.) ;
#22627=ORIENTED_EDGE('',*,*,#16609,.F.) ;
#22628=ORIENTED_EDGE('',*,*,#16539,.T.) ;
#22629=ORIENTED_EDGE('',*,*,#16610,.F.) ;
#22630=ORIENTED_EDGE('',*,*,#16611,.F.) ;
#22631=ORIENTED_EDGE('',*,*,#16612,.F.) ;
#22632=ORIENTED_EDGE('',*,*,#16552,.T.) ;
#22633=ORIENTED_EDGE('',*,*,#16573,.T.) ;
#22634=ORIENTED_EDGE('',*,*,#16592,.T.) ;
#22635=ORIENTED_EDGE('',*,*,#16613,.T.) ;
#22636=ORIENTED_EDGE('',*,*,#16614,.T.) ;
#22637=ORIENTED_EDGE('',*,*,#16602,.T.) ;
#22638=ORIENTED_EDGE('',*,*,#16615,.F.) ;
#22639=ORIENTED_EDGE('',*,*,#16616,.T.) ;
#22640=ORIENTED_EDGE('',*,*,#16591,.T.) ;
#22641=ORIENTED_EDGE('',*,*,#16617,.F.) ;
#22642=ORIENTED_EDGE('',*,*,#16618,.F.) ;
#22643=ORIENTED_EDGE('',*,*,#16613,.F.) ;
#22644=ORIENTED_EDGE('',*,*,#16553,.T.) ;
#22645=ORIENTED_EDGE('',*,*,#16616,.F.) ;
#22646=ORIENTED_EDGE('',*,*,#16619,.F.) ;
#22647=ORIENTED_EDGE('',*,*,#16620,.F.) ;
#22648=ORIENTED_EDGE('',*,*,#16531,.T.) ;
#22649=ORIENTED_EDGE('',*,*,#16565,.T.) ;
#22650=ORIENTED_EDGE('',*,*,#16577,.T.) ;
#22651=ORIENTED_EDGE('',*,*,#16621,.F.) ;
#22652=ORIENTED_EDGE('',*,*,#16622,.F.) ;
#22653=ORIENTED_EDGE('',*,*,#16623,.F.) ;
#22654=ORIENTED_EDGE('',*,*,#16624,.F.) ;
#22655=ORIENTED_EDGE('',*,*,#16625,.F.) ;
#22656=ORIENTED_EDGE('',*,*,#16579,.T.) ;
#22657=ORIENTED_EDGE('',*,*,#16626,.F.) ;
#22658=ORIENTED_EDGE('',*,*,#16627,.F.) ;
#22659=ORIENTED_EDGE('',*,*,#16628,.F.) ;
#22660=ORIENTED_EDGE('',*,*,#16547,.T.) ;
#22661=ORIENTED_EDGE('',*,*,#16561,.T.) ;
#22662=ORIENTED_EDGE('',*,*,#16588,.T.) ;
#22663=ORIENTED_EDGE('',*,*,#16629,.F.) ;
#22664=ORIENTED_EDGE('',*,*,#16630,.F.) ;
#22665=ORIENTED_EDGE('',*,*,#16631,.F.) ;
#22666=ORIENTED_EDGE('',*,*,#16632,.F.) ;
#22667=ORIENTED_EDGE('',*,*,#16633,.F.) ;
#22668=ORIENTED_EDGE('',*,*,#16586,.T.) ;
#22669=ORIENTED_EDGE('',*,*,#16634,.F.) ;
#22670=ORIENTED_EDGE('',*,*,#16635,.F.) ;
#22671=ORIENTED_EDGE('',*,*,#16636,.F.) ;
#22672=ORIENTED_EDGE('',*,*,#16549,.T.) ;
#22673=ORIENTED_EDGE('',*,*,#16637,.F.) ;
#22674=ORIENTED_EDGE('',*,*,#16638,.F.) ;
#22675=ORIENTED_EDGE('',*,*,#16639,.F.) ;
#22676=ORIENTED_EDGE('',*,*,#16543,.T.) ;
#22677=ORIENTED_EDGE('',*,*,#16564,.T.) ;
#22678=ORIENTED_EDGE('',*,*,#16584,.T.) ;
#22679=ORIENTED_EDGE('',*,*,#16640,.F.) ;
#22680=ORIENTED_EDGE('',*,*,#16641,.F.) ;
#22681=ORIENTED_EDGE('',*,*,#16642,.F.) ;
#22682=ORIENTED_EDGE('',*,*,#16643,.F.) ;
#22683=ORIENTED_EDGE('',*,*,#16644,.F.) ;
#22684=ORIENTED_EDGE('',*,*,#16544,.T.) ;
#22685=ORIENTED_EDGE('',*,*,#16644,.T.) ;
#22686=ORIENTED_EDGE('',*,*,#16645,.F.) ;
#22687=ORIENTED_EDGE('',*,*,#16646,.T.) ;
#22688=ORIENTED_EDGE('',*,*,#16548,.T.) ;
#22689=ORIENTED_EDGE('',*,*,#16633,.T.) ;
#22690=ORIENTED_EDGE('',*,*,#16647,.F.) ;
#22691=ORIENTED_EDGE('',*,*,#16637,.T.) ;
#22692=ORIENTED_EDGE('',*,*,#16554,.T.) ;
#22693=ORIENTED_EDGE('',*,*,#16620,.T.) ;
#22694=ORIENTED_EDGE('',*,*,#16648,.F.) ;
#22695=ORIENTED_EDGE('',*,*,#16649,.T.) ;
#22696=ORIENTED_EDGE('',*,*,#16532,.T.) ;
#22697=ORIENTED_EDGE('',*,*,#16625,.T.) ;
#22698=ORIENTED_EDGE('',*,*,#16650,.F.) ;
#22699=ORIENTED_EDGE('',*,*,#16651,.T.) ;
#22700=ORIENTED_EDGE('',*,*,#16540,.T.) ;
#22701=ORIENTED_EDGE('',*,*,#16612,.T.) ;
#22702=ORIENTED_EDGE('',*,*,#16652,.F.) ;
#22703=ORIENTED_EDGE('',*,*,#16605,.T.) ;
#22704=ORIENTED_EDGE('',*,*,#16558,.T.) ;
#22705=ORIENTED_EDGE('',*,*,#16653,.T.) ;
#22706=ORIENTED_EDGE('',*,*,#16654,.F.) ;
#22707=ORIENTED_EDGE('',*,*,#16600,.T.) ;
#22708=ORIENTED_EDGE('',*,*,#16655,.F.) ;
#22709=ORIENTED_EDGE('',*,*,#16603,.T.) ;
#22710=ORIENTED_EDGE('',*,*,#16614,.F.) ;
#22711=ORIENTED_EDGE('',*,*,#16618,.T.) ;
#22712=ORIENTED_EDGE('',*,*,#16619,.T.) ;
#22713=ORIENTED_EDGE('',*,*,#16615,.T.) ;
#22714=ORIENTED_EDGE('',*,*,#16601,.T.) ;
#22715=ORIENTED_EDGE('',*,*,#16654,.T.) ;
#22716=ORIENTED_EDGE('',*,*,#16656,.T.) ;
#22717=ORIENTED_EDGE('',*,*,#16657,.T.) ;
#22718=ORIENTED_EDGE('',*,*,#16658,.T.) ;
#22719=ORIENTED_EDGE('',*,*,#16650,.T.) ;
#22720=ORIENTED_EDGE('',*,*,#16624,.T.) ;
#22721=ORIENTED_EDGE('',*,*,#16659,.T.) ;
#22722=ORIENTED_EDGE('',*,*,#16606,.T.) ;
#22723=ORIENTED_EDGE('',*,*,#16652,.T.) ;
#22724=ORIENTED_EDGE('',*,*,#16611,.T.) ;
#22725=ORIENTED_EDGE('',*,*,#16660,.T.) ;
#22726=ORIENTED_EDGE('',*,*,#16661,.T.) ;
#22727=ORIENTED_EDGE('',*,*,#16645,.T.) ;
#22728=ORIENTED_EDGE('',*,*,#16643,.T.) ;
#22729=ORIENTED_EDGE('',*,*,#16662,.T.) ;
#22730=ORIENTED_EDGE('',*,*,#16638,.T.) ;
#22731=ORIENTED_EDGE('',*,*,#16647,.T.) ;
#22732=ORIENTED_EDGE('',*,*,#16632,.T.) ;
#22733=ORIENTED_EDGE('',*,*,#16663,.T.) ;
#22734=ORIENTED_EDGE('',*,*,#16664,.T.) ;
#22735=ORIENTED_EDGE('',*,*,#16648,.T.) ;
#22736=ORIENTED_EDGE('',*,*,#16599,.T.) ;
#22737=ORIENTED_EDGE('',*,*,#16665,.F.) ;
#22738=ORIENTED_EDGE('',*,*,#16666,.F.) ;
#22739=ORIENTED_EDGE('',*,*,#16667,.F.) ;
#22740=ORIENTED_EDGE('',*,*,#16656,.F.) ;
#22741=ORIENTED_EDGE('',*,*,#16653,.F.) ;
#22742=ORIENTED_EDGE('',*,*,#16557,.T.) ;
#22743=ORIENTED_EDGE('',*,*,#16576,.T.) ;
#22744=ORIENTED_EDGE('',*,*,#16533,.T.) ;
#22745=ORIENTED_EDGE('',*,*,#16651,.F.) ;
#22746=ORIENTED_EDGE('',*,*,#16658,.F.) ;
#22747=ORIENTED_EDGE('',*,*,#16668,.F.) ;
#22748=ORIENTED_EDGE('',*,*,#16534,.T.) ;
#22749=ORIENTED_EDGE('',*,*,#16668,.T.) ;
#22750=ORIENTED_EDGE('',*,*,#16657,.F.) ;
#22751=ORIENTED_EDGE('',*,*,#16667,.T.) ;
#22752=ORIENTED_EDGE('',*,*,#16669,.T.) ;
#22753=ORIENTED_EDGE('',*,*,#16626,.T.) ;
#22754=ORIENTED_EDGE('',*,*,#16578,.T.) ;
#22755=ORIENTED_EDGE('',*,*,#16566,.T.) ;
#22756=ORIENTED_EDGE('',*,*,#16670,.F.) ;
#22757=ORIENTED_EDGE('',*,*,#16627,.T.) ;
#22758=ORIENTED_EDGE('',*,*,#16669,.F.) ;
#22759=ORIENTED_EDGE('',*,*,#16666,.T.) ;
#22760=ORIENTED_EDGE('',*,*,#16671,.F.) ;
#22761=ORIENTED_EDGE('',*,*,#16608,.T.) ;
#22762=ORIENTED_EDGE('',*,*,#16672,.T.) ;
#22763=ORIENTED_EDGE('',*,*,#16622,.T.) ;
#22764=ORIENTED_EDGE('',*,*,#16672,.F.) ;
#22765=ORIENTED_EDGE('',*,*,#16607,.T.) ;
#22766=ORIENTED_EDGE('',*,*,#16659,.F.) ;
#22767=ORIENTED_EDGE('',*,*,#16623,.T.) ;
#22768=ORIENTED_EDGE('',*,*,#16673,.F.) ;
#22769=ORIENTED_EDGE('',*,*,#16674,.T.) ;
#22770=ORIENTED_EDGE('',*,*,#16582,.T.) ;
#22771=ORIENTED_EDGE('',*,*,#16675,.T.) ;
#22772=ORIENTED_EDGE('',*,*,#16676,.T.) ;
#22773=ORIENTED_EDGE('',*,*,#16677,.T.) ;
#22774=ORIENTED_EDGE('',*,*,#16594,.T.) ;
#22775=ORIENTED_EDGE('',*,*,#16609,.T.) ;
#22776=ORIENTED_EDGE('',*,*,#16671,.T.) ;
#22777=ORIENTED_EDGE('',*,*,#16621,.T.) ;
#22778=ORIENTED_EDGE('',*,*,#16580,.T.) ;
#22779=ORIENTED_EDGE('',*,*,#16628,.T.) ;
#22780=ORIENTED_EDGE('',*,*,#16670,.T.) ;
#22781=ORIENTED_EDGE('',*,*,#16665,.T.) ;
#22782=ORIENTED_EDGE('',*,*,#16598,.T.) ;
#22783=ORIENTED_EDGE('',*,*,#16604,.T.) ;
#22784=ORIENTED_EDGE('',*,*,#16655,.T.) ;
#22785=ORIENTED_EDGE('',*,*,#16617,.T.) ;
#22786=ORIENTED_EDGE('',*,*,#16590,.T.) ;
#22787=ORIENTED_EDGE('',*,*,#16678,.T.) ;
#22788=ORIENTED_EDGE('',*,*,#16679,.T.) ;
#22789=ORIENTED_EDGE('',*,*,#16629,.T.) ;
#22790=ORIENTED_EDGE('',*,*,#16587,.T.) ;
#22791=ORIENTED_EDGE('',*,*,#16636,.T.) ;
#22792=ORIENTED_EDGE('',*,*,#16680,.T.) ;
#22793=ORIENTED_EDGE('',*,*,#16640,.T.) ;
#22794=ORIENTED_EDGE('',*,*,#16583,.T.) ;
#22795=ORIENTED_EDGE('',*,*,#16674,.F.) ;
#22796=ORIENTED_EDGE('',*,*,#16595,.T.) ;
#22797=ORIENTED_EDGE('',*,*,#16677,.F.) ;
#22798=ORIENTED_EDGE('',*,*,#16681,.F.) ;
#22799=ORIENTED_EDGE('',*,*,#16682,.F.) ;
#22800=ORIENTED_EDGE('',*,*,#16541,.T.) ;
#22801=ORIENTED_EDGE('',*,*,#16646,.F.) ;
#22802=ORIENTED_EDGE('',*,*,#16661,.F.) ;
#22803=ORIENTED_EDGE('',*,*,#16683,.F.) ;
#22804=ORIENTED_EDGE('',*,*,#16684,.F.) ;
#22805=ORIENTED_EDGE('',*,*,#16675,.F.) ;
#22806=ORIENTED_EDGE('',*,*,#16581,.T.) ;
#22807=ORIENTED_EDGE('',*,*,#16562,.T.) ;
#22808=ORIENTED_EDGE('',*,*,#16596,.T.) ;
#22809=ORIENTED_EDGE('',*,*,#16682,.T.) ;
#22810=ORIENTED_EDGE('',*,*,#16685,.T.) ;
#22811=ORIENTED_EDGE('',*,*,#16683,.T.) ;
#22812=ORIENTED_EDGE('',*,*,#16660,.F.) ;
#22813=ORIENTED_EDGE('',*,*,#16610,.T.) ;
#22814=ORIENTED_EDGE('',*,*,#16538,.T.) ;
#22815=ORIENTED_EDGE('',*,*,#16570,.T.) ;
#22816=ORIENTED_EDGE('',*,*,#16676,.F.) ;
#22817=ORIENTED_EDGE('',*,*,#16684,.T.) ;
#22818=ORIENTED_EDGE('',*,*,#16685,.F.) ;
#22819=ORIENTED_EDGE('',*,*,#16681,.T.) ;
#22820=ORIENTED_EDGE('',*,*,#16545,.T.) ;
#22821=ORIENTED_EDGE('',*,*,#16639,.T.) ;
#22822=ORIENTED_EDGE('',*,*,#16662,.F.) ;
#22823=ORIENTED_EDGE('',*,*,#16642,.T.) ;
#22824=ORIENTED_EDGE('',*,*,#16686,.T.) ;
#22825=ORIENTED_EDGE('',*,*,#16634,.T.) ;
#22826=ORIENTED_EDGE('',*,*,#16585,.T.) ;
#22827=ORIENTED_EDGE('',*,*,#16559,.T.) ;
#22828=ORIENTED_EDGE('',*,*,#16680,.F.) ;
#22829=ORIENTED_EDGE('',*,*,#16635,.T.) ;
#22830=ORIENTED_EDGE('',*,*,#16686,.F.) ;
#22831=ORIENTED_EDGE('',*,*,#16641,.T.) ;
#22832=ORIENTED_EDGE('',*,*,#16550,.T.) ;
#22833=ORIENTED_EDGE('',*,*,#16649,.F.) ;
#22834=ORIENTED_EDGE('',*,*,#16664,.F.) ;
#22835=ORIENTED_EDGE('',*,*,#16687,.F.) ;
#22836=ORIENTED_EDGE('',*,*,#16688,.F.) ;
#22837=ORIENTED_EDGE('',*,*,#16678,.F.) ;
#22838=ORIENTED_EDGE('',*,*,#16589,.T.) ;
#22839=ORIENTED_EDGE('',*,*,#16571,.T.) ;
#22840=ORIENTED_EDGE('',*,*,#16663,.F.) ;
#22841=ORIENTED_EDGE('',*,*,#16631,.T.) ;
#22842=ORIENTED_EDGE('',*,*,#16689,.T.) ;
#22843=ORIENTED_EDGE('',*,*,#16687,.T.) ;
#22844=ORIENTED_EDGE('',*,*,#16679,.F.) ;
#22845=ORIENTED_EDGE('',*,*,#16688,.T.) ;
#22846=ORIENTED_EDGE('',*,*,#16689,.F.) ;
#22847=ORIENTED_EDGE('',*,*,#16630,.T.) ;
#22848=ORIENTED_EDGE('',*,*,#16690,.F.) ;
#22849=ORIENTED_EDGE('',*,*,#16691,.T.) ;
#22850=ORIENTED_EDGE('',*,*,#16692,.F.) ;
#22851=ORIENTED_EDGE('',*,*,#16691,.F.) ;
#22852=ORIENTED_EDGE('',*,*,#16690,.T.) ;
#22853=ORIENTED_EDGE('',*,*,#16693,.T.) ;
#22854=ORIENTED_EDGE('',*,*,#16673,.T.) ;
#22855=ORIENTED_EDGE('',*,*,#16694,.F.) ;
#22856=ORIENTED_EDGE('',*,*,#16695,.T.) ;
#22857=ORIENTED_EDGE('',*,*,#16693,.F.) ;
#22858=ORIENTED_EDGE('',*,*,#16695,.F.) ;
#22859=ORIENTED_EDGE('',*,*,#16694,.T.) ;
#22860=ORIENTED_EDGE('',*,*,#16692,.T.) ;
#26802=CYLINDRICAL_SURFACE('',#30426,1.55) ;
#26803=CYLINDRICAL_SURFACE('',#30428,1.55) ;
#26804=CYLINDRICAL_SURFACE('',#30430,1.55) ;
#26805=CYLINDRICAL_SURFACE('',#30432,1.55) ;
#26806=CYLINDRICAL_SURFACE('',#30434,1.55) ;
#26807=CYLINDRICAL_SURFACE('',#30436,1.55) ;
#26808=CYLINDRICAL_SURFACE('',#30463,1.75) ;
#26809=CYLINDRICAL_SURFACE('',#30465,1.75) ;
#26810=CYLINDRICAL_SURFACE('',#30467,1.75) ;
#26811=CYLINDRICAL_SURFACE('',#30469,1.75) ;
#26812=CYLINDRICAL_SURFACE('',#30471,1.75) ;
#26813=CYLINDRICAL_SURFACE('',#30473,1.75) ;
#26814=CYLINDRICAL_SURFACE('',#30486,1.75) ;
#26815=CYLINDRICAL_SURFACE('',#30500,1.75) ;
#26816=CYLINDRICAL_SURFACE('',#30506,2.2) ;
#27836=ADVANCED_FACE('',(#3101),#1988,.F.) ;
#27837=ADVANCED_FACE('',(#3102),#1989,.F.) ;
#27838=ADVANCED_FACE('',(#3103),#1990,.F.) ;
#27839=ADVANCED_FACE('',(#3104),#1991,.F.) ;
#27840=ADVANCED_FACE('',(#3105),#1992,.F.) ;
#27841=ADVANCED_FACE('',(#3106),#1993,.F.) ;
#27842=ADVANCED_FACE('',(#3107),#26802,.T.) ;
#27843=ADVANCED_FACE('',(#3108),#26803,.T.) ;
#27844=ADVANCED_FACE('',(#3109),#26804,.T.) ;
#27845=ADVANCED_FACE('',(#3110),#26805,.T.) ;
#27846=ADVANCED_FACE('',(#3111),#26806,.T.) ;
#27847=ADVANCED_FACE('',(#3112),#26807,.T.) ;
#27848=ADVANCED_FACE('',(#3113),#1994,.F.) ;
#27849=ADVANCED_FACE('',(#3114),#1995,.F.) ;
#27850=ADVANCED_FACE('',(#3115),#1996,.F.) ;
#27851=ADVANCED_FACE('',(#3116),#1997,.F.) ;
#27852=ADVANCED_FACE('',(#3117),#1998,.F.) ;
#27853=ADVANCED_FACE('',(#3118),#1999,.F.) ;
#27854=ADVANCED_FACE('',(#3119),#2000,.T.) ;
#27855=ADVANCED_FACE('',(#3120),#2001,.F.) ;
#27856=ADVANCED_FACE('',(#3121),#2002,.F.) ;
#27857=ADVANCED_FACE('',(#3122),#2003,.T.) ;
#27858=ADVANCED_FACE('',(#3123),#2004,.F.) ;
#27859=ADVANCED_FACE('',(#3124),#2005,.F.) ;
#27860=ADVANCED_FACE('',(#3125),#2006,.T.) ;
#27861=ADVANCED_FACE('',(#3126),#2007,.T.) ;
#27862=ADVANCED_FACE('',(#3127),#2008,.F.) ;
#27863=ADVANCED_FACE('',(#3128),#2009,.T.) ;
#27864=ADVANCED_FACE('',(#3129),#2010,.T.) ;
#27865=ADVANCED_FACE('',(#3130),#2011,.F.) ;
#27866=ADVANCED_FACE('',(#3131),#26808,.T.) ;
#27867=ADVANCED_FACE('',(#3132),#26809,.T.) ;
#27868=ADVANCED_FACE('',(#3133),#26810,.T.) ;
#27869=ADVANCED_FACE('',(#3134),#26811,.T.) ;
#27870=ADVANCED_FACE('',(#3135),#26812,.T.) ;
#27871=ADVANCED_FACE('',(#3136),#26813,.T.) ;
#27872=ADVANCED_FACE('',(#3137),#2012,.T.) ;
#27873=ADVANCED_FACE('',(#3138),#2013,.T.) ;
#27874=ADVANCED_FACE('',(#3139),#2014,.F.) ;
#27875=ADVANCED_FACE('',(#3140),#2015,.T.) ;
#27876=ADVANCED_FACE('',(#3141),#2016,.T.) ;
#27877=ADVANCED_FACE('',(#3142),#2017,.T.) ;
#27878=ADVANCED_FACE('',(#3143),#2018,.T.) ;
#27879=ADVANCED_FACE('',(#3144),#2019,.T.) ;
#27880=ADVANCED_FACE('',(#3145),#26814,.T.) ;
#27881=ADVANCED_FACE('',(#3146),#2020,.F.) ;
#27882=ADVANCED_FACE('',(#3147),#2021,.T.) ;
#27883=ADVANCED_FACE('',(#3148),#2022,.T.) ;
#27884=ADVANCED_FACE('',(#3149),#2023,.T.) ;
#27885=ADVANCED_FACE('',(#3150),#2024,.T.) ;
#27886=ADVANCED_FACE('',(#3151),#2025,.T.) ;
#27887=ADVANCED_FACE('',(#3152),#2026,.T.) ;
#27888=ADVANCED_FACE('',(#3153),#2027,.T.) ;
#27889=ADVANCED_FACE('',(#3154),#2028,.T.) ;
#27890=ADVANCED_FACE('',(#3155),#26815,.T.) ;
#27891=ADVANCED_FACE('',(#3156),#2029,.T.) ;
#27892=ADVANCED_FACE('',(#3157,#1295),#2030,.T.) ;
#27893=ADVANCED_FACE('',(#3158),#26816,.T.) ;
#27894=ADVANCED_FACE('',(#3159,#1296),#2031,.T.) ;
#28659=CLOSED_SHELL('',(#27836,#27837,#27838,#27839,#27840,#27841,#27842,
#27843,#27844,#27845,#27846,#27847,#27848,#27849,#27850,#27851,#27852,#27853,
#27854,#27855,#27856,#27857,#27858,#27859,#27860,#27861,#27862,#27863,#27864,
#27865,#27866,#27867,#27868,#27869,#27870,#27871,#27872,#27873,#27874,#27875,
#27876,#27877,#27878,#27879,#27880,#27881,#27882,#27883,#27884,#27885,#27886,
#27887,#27888,#27889,#27890,#27891,#27892,#27893,#27894)) ;
#30407=AXIS2_PLACEMENT_3D('',#45457,#36323,#36324) ;
#30408=AXIS2_PLACEMENT_3D('',#45458,#36325,#36326) ;
#30409=AXIS2_PLACEMENT_3D('',#45463,#36328,#36329) ;
#30410=AXIS2_PLACEMENT_3D('',#45468,#36332,#36333) ;
#30411=AXIS2_PLACEMENT_3D('',#45469,#36334,#36335) ;
#30412=AXIS2_PLACEMENT_3D('',#45474,#36337,#36338) ;
#30413=AXIS2_PLACEMENT_3D('',#45479,#36341,#36342) ;
#30414=AXIS2_PLACEMENT_3D('',#45480,#36343,#36344) ;
#30415=AXIS2_PLACEMENT_3D('',#45485,#36346,#36347) ;
#30416=AXIS2_PLACEMENT_3D('',#45488,#36349,#36350) ;
#30417=AXIS2_PLACEMENT_3D('',#45489,#36351,#36352) ;
#30418=AXIS2_PLACEMENT_3D('',#45494,#36354,#36355) ;
#30419=AXIS2_PLACEMENT_3D('',#45498,#36357,#36358) ;
#30420=AXIS2_PLACEMENT_3D('',#45500,#36360,#36361) ;
#30421=AXIS2_PLACEMENT_3D('',#45505,#36363,#36364) ;
#30422=AXIS2_PLACEMENT_3D('',#45510,#36367,#36368) ;
#30423=AXIS2_PLACEMENT_3D('',#45511,#36369,#36370) ;
#30424=AXIS2_PLACEMENT_3D('',#45516,#36372,#36373) ;
#30425=AXIS2_PLACEMENT_3D('',#45519,#36375,#36376) ;
#30426=AXIS2_PLACEMENT_3D('',#45520,#36377,#36378) ;
#30427=AXIS2_PLACEMENT_3D('',#45524,#36380,#36381) ;
#30428=AXIS2_PLACEMENT_3D('',#45526,#36383,#36384) ;
#30429=AXIS2_PLACEMENT_3D('',#45530,#36386,#36387) ;
#30430=AXIS2_PLACEMENT_3D('',#45532,#36389,#36390) ;
#30431=AXIS2_PLACEMENT_3D('',#45537,#36393,#36394) ;
#30432=AXIS2_PLACEMENT_3D('',#45538,#36395,#36396) ;
#30433=AXIS2_PLACEMENT_3D('',#45542,#36398,#36399) ;
#30434=AXIS2_PLACEMENT_3D('',#45544,#36401,#36402) ;
#30435=AXIS2_PLACEMENT_3D('',#45548,#36404,#36405) ;
#30436=AXIS2_PLACEMENT_3D('',#45550,#36407,#36408) ;
#30437=AXIS2_PLACEMENT_3D('',#45554,#36410,#36411) ;
#30438=AXIS2_PLACEMENT_3D('',#45556,#36413,#36414) ;
#30439=AXIS2_PLACEMENT_3D('',#45563,#36418,#36419) ;
#30440=AXIS2_PLACEMENT_3D('',#45564,#36420,#36421) ;
#30441=AXIS2_PLACEMENT_3D('',#45568,#36423,#36424) ;
#30442=AXIS2_PLACEMENT_3D('',#45570,#36425,#36426) ;
#30443=AXIS2_PLACEMENT_3D('',#45572,#36428,#36429) ;
#30444=AXIS2_PLACEMENT_3D('',#45578,#36432,#36433) ;
#30445=AXIS2_PLACEMENT_3D('',#45580,#36435,#36436) ;
#30446=AXIS2_PLACEMENT_3D('',#45584,#36438,#36439) ;
#30447=AXIS2_PLACEMENT_3D('',#45588,#36442,#36443) ;
#30448=AXIS2_PLACEMENT_3D('',#45592,#36445,#36446) ;
#30449=AXIS2_PLACEMENT_3D('',#45596,#36449,#36450) ;
#30450=AXIS2_PLACEMENT_3D('',#45600,#36452,#36453) ;
#30451=AXIS2_PLACEMENT_3D('',#45602,#36455,#36456) ;
#30452=AXIS2_PLACEMENT_3D('',#45612,#36462,#36463) ;
#30453=AXIS2_PLACEMENT_3D('',#45622,#36469,#36470) ;
#30454=AXIS2_PLACEMENT_3D('',#45628,#36474,#36475) ;
#30455=AXIS2_PLACEMENT_3D('',#45635,#36480,#36481) ;
#30456=AXIS2_PLACEMENT_3D('',#45639,#36484,#36485) ;
#30457=AXIS2_PLACEMENT_3D('',#45643,#36488,#36489) ;
#30458=AXIS2_PLACEMENT_3D('',#45653,#36495,#36496) ;
#30459=AXIS2_PLACEMENT_3D('',#45659,#36500,#36501) ;
#30460=AXIS2_PLACEMENT_3D('',#45669,#36507,#36508) ;
#30461=AXIS2_PLACEMENT_3D('',#45675,#36512,#36513) ;
#30462=AXIS2_PLACEMENT_3D('',#45681,#36517,#36518) ;
#30463=AXIS2_PLACEMENT_3D('',#45691,#36524,#36525) ;
#30464=AXIS2_PLACEMENT_3D('',#45693,#36526,#36527) ;
#30465=AXIS2_PLACEMENT_3D('',#45695,#36529,#36530) ;
#30466=AXIS2_PLACEMENT_3D('',#45696,#36531,#36532) ;
#30467=AXIS2_PLACEMENT_3D('',#45697,#36533,#36534) ;
#30468=AXIS2_PLACEMENT_3D('',#45699,#36535,#36536) ;
#30469=AXIS2_PLACEMENT_3D('',#45701,#36538,#36539) ;
#30470=AXIS2_PLACEMENT_3D('',#45703,#36540,#36541) ;
#30471=AXIS2_PLACEMENT_3D('',#45705,#36543,#36544) ;
#30472=AXIS2_PLACEMENT_3D('',#45706,#36545,#36546) ;
#30473=AXIS2_PLACEMENT_3D('',#45707,#36547,#36548) ;
#30474=AXIS2_PLACEMENT_3D('',#45710,#36550,#36551) ;
#30475=AXIS2_PLACEMENT_3D('',#45711,#36552,#36553) ;
#30476=AXIS2_PLACEMENT_3D('',#45712,#36554,#36555) ;
#30477=AXIS2_PLACEMENT_3D('',#45713,#36556,#36557) ;
#30478=AXIS2_PLACEMENT_3D('',#45727,#36567,#36568) ;
#30479=AXIS2_PLACEMENT_3D('',#45733,#36572,#36573) ;
#30480=AXIS2_PLACEMENT_3D('',#45735,#36575,#36576) ;
#30481=AXIS2_PLACEMENT_3D('',#45737,#36578,#36579) ;
#30482=AXIS2_PLACEMENT_3D('',#45738,#36580,#36581) ;
#30483=AXIS2_PLACEMENT_3D('',#45739,#36582,#36583) ;
#30484=AXIS2_PLACEMENT_3D('',#45740,#36584,#36585) ;
#30485=AXIS2_PLACEMENT_3D('',#45742,#36587,#36588) ;
#30486=AXIS2_PLACEMENT_3D('',#45743,#36589,#36590) ;
#30487=AXIS2_PLACEMENT_3D('',#45745,#36591,#36592) ;
#30488=AXIS2_PLACEMENT_3D('',#45750,#36595,#36596) ;
#30489=AXIS2_PLACEMENT_3D('',#45754,#36599,#36600) ;
#30490=AXIS2_PLACEMENT_3D('',#45755,#36601,#36602) ;
#30491=AXIS2_PLACEMENT_3D('',#45756,#36603,#36604) ;
#30492=AXIS2_PLACEMENT_3D('',#45760,#36607,#36608) ;
#30493=AXIS2_PLACEMENT_3D('',#45764,#36611,#36612) ;
#30494=AXIS2_PLACEMENT_3D('',#45766,#36614,#36615) ;
#30495=AXIS2_PLACEMENT_3D('',#45767,#36616,#36617) ;
#30496=AXIS2_PLACEMENT_3D('',#45769,#36619,#36620) ;
#30497=AXIS2_PLACEMENT_3D('',#45770,#36621,#36622) ;
#30498=AXIS2_PLACEMENT_3D('',#45774,#36625,#36626) ;
#30499=AXIS2_PLACEMENT_3D('',#45776,#36628,#36629) ;
#30500=AXIS2_PLACEMENT_3D('',#45777,#36630,#36631) ;
#30501=AXIS2_PLACEMENT_3D('',#45779,#36632,#36633) ;
#30502=AXIS2_PLACEMENT_3D('',#45782,#36635,#36636) ;
#30503=AXIS2_PLACEMENT_3D('',#45783,#36637,#36638) ;
#30504=AXIS2_PLACEMENT_3D('',#45784,#36639,#36640) ;
#30505=AXIS2_PLACEMENT_3D('',#45786,#36641,#36642) ;
#30506=AXIS2_PLACEMENT_3D('',#45787,#36643,#36644) ;
#30507=AXIS2_PLACEMENT_3D('',#45789,#36645,#36646) ;
#30508=AXIS2_PLACEMENT_3D('',#45791,#36648,#36649) ;
#36323=DIRECTION('axis',(0.,0.,1.)) ;
#36324=DIRECTION('refdir',(1.,0.,0.)) ;
#36325=DIRECTION('center_axis',(-1.,0.,0.)) ;
#36326=DIRECTION('ref_axis',(0.,0.,1.)) ;
#36327=DIRECTION('',(0.,1.,0.)) ;
#36328=DIRECTION('center_axis',(-1.,0.,0.)) ;
#36329=DIRECTION('ref_axis',(0.,0.,-1.)) ;
#36330=DIRECTION('',(0.,0.,-1.)) ;
#36331=DIRECTION('',(0.,-1.,0.)) ;
#36332=DIRECTION('center_axis',(1.,0.,0.)) ;
#36333=DIRECTION('ref_axis',(0.,0.,-1.)) ;
#36334=DIRECTION('center_axis',(-1.,0.,0.)) ;
#36335=DIRECTION('ref_axis',(0.,0.,1.)) ;
#36336=DIRECTION('',(0.,-1.,0.)) ;
#36337=DIRECTION('center_axis',(1.,0.,0.)) ;
#36338=DIRECTION('ref_axis',(0.,0.,-1.)) ;
#36339=DIRECTION('',(0.,1.,0.)) ;
#36340=DIRECTION('',(0.,0.,-1.)) ;
#36341=DIRECTION('center_axis',(-1.,0.,0.)) ;
#36342=DIRECTION('ref_axis',(0.,0.,-1.)) ;
#36343=DIRECTION('center_axis',(-1.,0.,0.)) ;
#36344=DIRECTION('ref_axis',(0.,0.,1.)) ;
#36345=DIRECTION('',(0.,0.,1.)) ;
#36346=DIRECTION('center_axis',(1.,0.,0.)) ;
#36347=DIRECTION('ref_axis',(0.,0.,-1.)) ;
#36348=DIRECTION('',(0.,0.,-1.)) ;
#36349=DIRECTION('center_axis',(-1.,0.,0.)) ;
#36350=DIRECTION('ref_axis',(0.,0.,-1.)) ;
#36351=DIRECTION('center_axis',(-1.,0.,0.)) ;
#36352=DIRECTION('ref_axis',(0.,0.,1.)) ;
#36353=DIRECTION('',(0.,1.,0.)) ;
#36354=DIRECTION('center_axis',(1.,0.,0.)) ;
#36355=DIRECTION('ref_axis',(0.,0.,-1.)) ;
#36356=DIRECTION('',(0.,-1.,0.)) ;
#36357=DIRECTION('center_axis',(-1.,0.,0.)) ;
#36358=DIRECTION('ref_axis',(0.,0.,-1.)) ;
#36359=DIRECTION('',(0.,0.,1.)) ;
#36360=DIRECTION('center_axis',(-1.,0.,0.)) ;
#36361=DIRECTION('ref_axis',(0.,0.,1.)) ;
#36362=DIRECTION('',(0.,1.,0.)) ;
#36363=DIRECTION('center_axis',(1.,0.,0.)) ;
#36364=DIRECTION('ref_axis',(0.,0.,-1.)) ;
#36365=DIRECTION('',(0.,-1.,0.)) ;
#36366=DIRECTION('',(0.,0.,1.)) ;
#36367=DIRECTION('center_axis',(-1.,0.,0.)) ;
#36368=DIRECTION('ref_axis',(0.,0.,-1.)) ;
#36369=DIRECTION('center_axis',(-1.,0.,0.)) ;
#36370=DIRECTION('ref_axis',(0.,0.,1.)) ;
#36371=DIRECTION('',(0.,0.,-1.)) ;
#36372=DIRECTION('center_axis',(1.,0.,0.)) ;
#36373=DIRECTION('ref_axis',(0.,0.,-1.)) ;
#36374=DIRECTION('',(0.,0.,1.)) ;
#36375=DIRECTION('center_axis',(-1.,0.,0.)) ;
#36376=DIRECTION('ref_axis',(0.,0.,-1.)) ;
#36377=DIRECTION('center_axis',(1.,0.,0.)) ;
#36378=DIRECTION('ref_axis',(0.,0.,-1.)) ;
#36379=DIRECTION('',(-1.,0.,0.)) ;
#36380=DIRECTION('center_axis',(-1.,0.,0.)) ;
#36381=DIRECTION('ref_axis',(0.,0.,-1.)) ;
#36382=DIRECTION('',(1.,0.,0.)) ;
#36383=DIRECTION('center_axis',(1.,0.,0.)) ;
#36384=DIRECTION('ref_axis',(0.,-1.22464679914735E-16,1.)) ;
#36385=DIRECTION('',(-1.,0.,0.)) ;
#36386=DIRECTION('center_axis',(-1.,0.,0.)) ;
#36387=DIRECTION('ref_axis',(0.,0.,-1.)) ;
#36388=DIRECTION('',(1.,0.,0.)) ;
#36389=DIRECTION('center_axis',(1.,0.,0.)) ;
#36390=DIRECTION('ref_axis',(0.,0.,-1.)) ;
#36391=DIRECTION('',(1.,0.,0.)) ;
#36392=DIRECTION('',(-1.,0.,0.)) ;
#36393=DIRECTION('center_axis',(-1.,0.,0.)) ;
#36394=DIRECTION('ref_axis',(0.,0.,-1.)) ;
#36395=DIRECTION('center_axis',(1.,0.,0.)) ;
#36396=DIRECTION('ref_axis',(0.,0.,-1.)) ;
#36397=DIRECTION('',(-1.,0.,0.)) ;
#36398=DIRECTION('center_axis',(-1.,0.,0.)) ;
#36399=DIRECTION('ref_axis',(0.,0.,-1.)) ;
#36400=DIRECTION('',(1.,0.,0.)) ;
#36401=DIRECTION('center_axis',(1.,0.,0.)) ;
#36402=DIRECTION('ref_axis',(0.,0.,-1.)) ;
#36403=DIRECTION('',(-1.,0.,0.)) ;
#36404=DIRECTION('center_axis',(-1.,0.,0.)) ;
#36405=DIRECTION('ref_axis',(0.,0.,-1.)) ;
#36406=DIRECTION('',(1.,0.,0.)) ;
#36407=DIRECTION('center_axis',(1.,0.,0.)) ;
#36408=DIRECTION('ref_axis',(0.,0.,-1.)) ;
#36409=DIRECTION('',(-1.,0.,0.)) ;
#36410=DIRECTION('center_axis',(-1.,0.,0.)) ;
#36411=DIRECTION('ref_axis',(0.,0.,-1.)) ;
#36412=DIRECTION('',(1.,0.,0.)) ;
#36413=DIRECTION('center_axis',(1.,0.,0.)) ;
#36414=DIRECTION('ref_axis',(0.,0.,-1.)) ;
#36415=DIRECTION('',(0.,-1.,0.)) ;
#36416=DIRECTION('',(0.,1.,0.)) ;
#36417=DIRECTION('',(0.,0.,1.)) ;
#36418=DIRECTION('center_axis',(1.,0.,0.)) ;
#36419=DIRECTION('ref_axis',(0.,0.,-1.)) ;
#36420=DIRECTION('center_axis',(1.,0.,0.)) ;
#36421=DIRECTION('ref_axis',(0.,0.,-1.)) ;
#36422=DIRECTION('',(0.,0.,-1.)) ;
#36423=DIRECTION('center_axis',(1.,0.,0.)) ;
#36424=DIRECTION('ref_axis',(0.,0.,-1.)) ;
#36425=DIRECTION('center_axis',(1.,0.,0.)) ;
#36426=DIRECTION('ref_axis',(0.,0.,-1.)) ;
#36427=DIRECTION('',(0.,0.,1.)) ;
#36428=DIRECTION('center_axis',(1.,0.,0.)) ;
#36429=DIRECTION('ref_axis',(0.,0.,-1.)) ;
#36430=DIRECTION('',(0.,-1.,0.)) ;
#36431=DIRECTION('',(0.,0.,-1.)) ;
#36432=DIRECTION('center_axis',(1.,0.,0.)) ;
#36433=DIRECTION('ref_axis',(0.,0.,-1.)) ;
#36434=DIRECTION('',(0.,1.,0.)) ;
#36435=DIRECTION('center_axis',(1.,0.,0.)) ;
#36436=DIRECTION('ref_axis',(0.,0.,-1.)) ;
#36437=DIRECTION('',(0.,-1.,0.)) ;
#36438=DIRECTION('center_axis',(1.,0.,0.)) ;
#36439=DIRECTION('ref_axis',(0.,0.,-1.)) ;
#36440=DIRECTION('',(0.,0.,-1.)) ;
#36441=DIRECTION('',(0.,1.,0.)) ;
#36442=DIRECTION('center_axis',(1.,0.,0.)) ;
#36443=DIRECTION('ref_axis',(0.,0.,-1.)) ;
#36444=DIRECTION('',(0.,1.,0.)) ;
#36445=DIRECTION('center_axis',(1.,0.,0.)) ;
#36446=DIRECTION('ref_axis',(0.,0.,-1.)) ;
#36447=DIRECTION('',(0.,0.,1.)) ;
#36448=DIRECTION('',(0.,-1.,0.)) ;
#36449=DIRECTION('center_axis',(1.,0.,0.)) ;
#36450=DIRECTION('ref_axis',(0.,0.,-1.)) ;
#36451=DIRECTION('',(0.,0.,1.)) ;
#36452=DIRECTION('center_axis',(1.,0.,0.)) ;
#36453=DIRECTION('ref_axis',(0.,0.,-1.)) ;
#36454=DIRECTION('',(0.,0.,-1.)) ;
#36455=DIRECTION('center_axis',(0.,1.,0.)) ;
#36456=DIRECTION('ref_axis',(1.,0.,0.)) ;
#36457=DIRECTION('',(1.,0.,0.)) ;
#36458=DIRECTION('',(0.,0.,-1.)) ;
#36459=DIRECTION('',(-1.,0.,0.)) ;
#36460=DIRECTION('',(0.,0.,1.)) ;
#36461=DIRECTION('',(1.,0.,0.)) ;
#36462=DIRECTION('center_axis',(0.,0.,1.)) ;
#36463=DIRECTION('ref_axis',(1.,0.,0.)) ;
#36464=DIRECTION('',(1.,0.,0.)) ;
#36465=DIRECTION('',(0.,-1.,0.)) ;
#36466=DIRECTION('',(-1.,0.,0.)) ;
#36467=DIRECTION('',(0.,1.,0.)) ;
#36468=DIRECTION('',(1.,0.,0.)) ;
#36469=DIRECTION('center_axis',(0.,-1.,0.)) ;
#36470=DIRECTION('ref_axis',(1.,0.,0.)) ;
#36471=DIRECTION('',(1.,0.,0.)) ;
#36472=DIRECTION('',(0.,0.,-1.)) ;
#36473=DIRECTION('',(-1.,0.,0.)) ;
#36474=DIRECTION('center_axis',(0.,0.,-1.)) ;
#36475=DIRECTION('ref_axis',(0.,1.,0.)) ;
#36476=DIRECTION('',(1.,0.,0.)) ;
#36477=DIRECTION('',(0.,-1.,0.)) ;
#36478=DIRECTION('',(0.,-1.,0.)) ;
#36479=DIRECTION('',(1.,0.,0.)) ;
#36480=DIRECTION('center_axis',(0.,1.,0.)) ;
#36481=DIRECTION('ref_axis',(1.,0.,0.)) ;
#36482=DIRECTION('',(-1.,0.,0.)) ;
#36483=DIRECTION('',(0.,0.,-1.)) ;
#36484=DIRECTION('center_axis',(0.,1.,0.)) ;
#36485=DIRECTION('ref_axis',(1.,0.,0.)) ;
#36486=DIRECTION('',(0.,0.,1.)) ;
#36487=DIRECTION('',(-1.,0.,0.)) ;
#36488=DIRECTION('center_axis',(0.,0.,1.)) ;
#36489=DIRECTION('ref_axis',(1.,0.,0.)) ;
#36490=DIRECTION('',(-1.,0.,0.)) ;
#36491=DIRECTION('',(0.,-1.,0.)) ;
#36492=DIRECTION('',(1.,0.,0.)) ;
#36493=DIRECTION('',(0.,1.,0.)) ;
#36494=DIRECTION('',(-1.,0.,0.)) ;
#36495=DIRECTION('center_axis',(0.,1.,0.)) ;
#36496=DIRECTION('ref_axis',(1.,0.,0.)) ;
#36497=DIRECTION('',(-1.,0.,0.)) ;
#36498=DIRECTION('',(0.,0.,1.)) ;
#36499=DIRECTION('',(1.,0.,0.)) ;
#36500=DIRECTION('center_axis',(0.,0.,1.)) ;
#36501=DIRECTION('ref_axis',(1.,0.,0.)) ;
#36502=DIRECTION('',(-1.,0.,0.)) ;
#36503=DIRECTION('',(0.,1.,0.)) ;
#36504=DIRECTION('',(1.,0.,0.)) ;
#36505=DIRECTION('',(0.,-1.,0.)) ;
#36506=DIRECTION('',(-1.,0.,0.)) ;
#36507=DIRECTION('center_axis',(0.,-1.,0.)) ;
#36508=DIRECTION('ref_axis',(1.,0.,0.)) ;
#36509=DIRECTION('',(-1.,0.,0.)) ;
#36510=DIRECTION('',(0.,0.,-1.)) ;
#36511=DIRECTION('',(1.,0.,0.)) ;
#36512=DIRECTION('center_axis',(0.,-1.,0.)) ;
#36513=DIRECTION('ref_axis',(1.,0.,0.)) ;
#36514=DIRECTION('',(1.,0.,0.)) ;
#36515=DIRECTION('',(0.,0.,1.)) ;
#36516=DIRECTION('',(-1.,0.,0.)) ;
#36517=DIRECTION('center_axis',(0.,-1.,0.)) ;
#36518=DIRECTION('ref_axis',(1.,0.,0.)) ;
#36519=DIRECTION('',(-1.,0.,0.)) ;
#36520=DIRECTION('',(0.,0.,1.)) ;
#36521=DIRECTION('',(1.,0.,0.)) ;
#36522=DIRECTION('',(0.,0.,-1.)) ;
#36523=DIRECTION('',(-1.,0.,0.)) ;
#36524=DIRECTION('center_axis',(1.,0.,0.)) ;
#36525=DIRECTION('ref_axis',(0.,1.22464679914735E-16,1.)) ;
#36526=DIRECTION('center_axis',(-1.,0.,0.)) ;
#36527=DIRECTION('ref_axis',(0.,0.,-1.)) ;
#36528=DIRECTION('',(1.,0.,0.)) ;
#36529=DIRECTION('center_axis',(1.,0.,0.)) ;
#36530=DIRECTION('ref_axis',(0.,0.,-1.)) ;
#36531=DIRECTION('center_axis',(-1.,0.,0.)) ;
#36532=DIRECTION('ref_axis',(0.,0.,-1.)) ;
#36533=DIRECTION('center_axis',(1.,0.,0.)) ;
#36534=DIRECTION('ref_axis',(0.,0.,-1.)) ;
#36535=DIRECTION('center_axis',(-1.,0.,0.)) ;
#36536=DIRECTION('ref_axis',(0.,0.,-1.)) ;
#36537=DIRECTION('',(1.,0.,0.)) ;
#36538=DIRECTION('center_axis',(1.,0.,0.)) ;
#36539=DIRECTION('ref_axis',(0.,0.,-1.)) ;
#36540=DIRECTION('center_axis',(-1.,0.,0.)) ;
#36541=DIRECTION('ref_axis',(0.,0.,-1.)) ;
#36542=DIRECTION('',(1.,0.,0.)) ;
#36543=DIRECTION('center_axis',(1.,0.,0.)) ;
#36544=DIRECTION('ref_axis',(0.,0.,-1.)) ;
#36545=DIRECTION('center_axis',(-1.,0.,0.)) ;
#36546=DIRECTION('ref_axis',(0.,0.,-1.)) ;
#36547=DIRECTION('center_axis',(1.,0.,0.)) ;
#36548=DIRECTION('ref_axis',(0.,0.,-1.)) ;
#36549=DIRECTION('',(-1.,0.,0.)) ;
#36550=DIRECTION('center_axis',(-1.,0.,0.)) ;
#36551=DIRECTION('ref_axis',(0.,0.,-1.)) ;
#36552=DIRECTION('center_axis',(-1.,0.,0.)) ;
#36553=DIRECTION('ref_axis',(0.,1.,0.)) ;
#36554=DIRECTION('center_axis',(1.,0.,0.)) ;
#36555=DIRECTION('ref_axis',(0.,0.,-1.)) ;
#36556=DIRECTION('center_axis',(-1.,0.,0.)) ;
#36557=DIRECTION('ref_axis',(0.,0.,1.)) ;
#36558=DIRECTION('',(0.,0.,1.)) ;
#36559=DIRECTION('',(0.,-1.,0.)) ;
#36560=DIRECTION('',(0.,0.,-1.)) ;
#36561=DIRECTION('',(0.,0.,1.)) ;
#36562=DIRECTION('',(0.,1.,0.)) ;
#36563=DIRECTION('',(0.,0.,1.)) ;
#36564=DIRECTION('',(0.,1.,0.)) ;
#36565=DIRECTION('',(0.,0.,-1.)) ;
#36566=DIRECTION('',(0.,1.,0.)) ;
#36567=DIRECTION('center_axis',(0.,1.,0.)) ;
#36568=DIRECTION('ref_axis',(1.,0.,0.)) ;
#36569=DIRECTION('',(-1.,0.,0.)) ;
#36570=DIRECTION('',(0.,0.,-1.)) ;
#36571=DIRECTION('',(1.,0.,0.)) ;
#36572=DIRECTION('center_axis',(0.,1.,0.)) ;
#36573=DIRECTION('ref_axis',(1.,0.,0.)) ;
#36574=DIRECTION('',(-1.,0.,0.)) ;
#36575=DIRECTION('center_axis',(0.,0.,-1.)) ;
#36576=DIRECTION('ref_axis',(0.,1.,0.)) ;
#36577=DIRECTION('',(0.,-1.,0.)) ;
#36578=DIRECTION('center_axis',(-1.,0.,0.)) ;
#36579=DIRECTION('ref_axis',(0.,1.,0.)) ;
#36580=DIRECTION('center_axis',(1.,0.,0.)) ;
#36581=DIRECTION('ref_axis',(0.,0.,-1.)) ;
#36582=DIRECTION('center_axis',(-1.,0.,0.)) ;
#36583=DIRECTION('ref_axis',(0.,0.,1.)) ;
#36584=DIRECTION('center_axis',(1.,0.,0.)) ;
#36585=DIRECTION('ref_axis',(0.,0.,-1.)) ;
#36586=DIRECTION('',(0.,0.,-1.)) ;
#36587=DIRECTION('center_axis',(0.,-1.,0.)) ;
#36588=DIRECTION('ref_axis',(0.,0.,-1.)) ;
#36589=DIRECTION('center_axis',(1.,0.,0.)) ;
#36590=DIRECTION('ref_axis',(0.,0.,-1.)) ;
#36591=DIRECTION('center_axis',(1.,0.,0.)) ;
#36592=DIRECTION('ref_axis',(0.,0.,-1.)) ;
#36593=DIRECTION('',(-1.,0.,0.)) ;
#36594=DIRECTION('',(1.,0.,0.)) ;
#36595=DIRECTION('center_axis',(1.,0.,0.)) ;
#36596=DIRECTION('ref_axis',(0.,0.,-1.)) ;
#36597=DIRECTION('',(-1.,0.,0.)) ;
#36598=DIRECTION('',(1.,0.,0.)) ;
#36599=DIRECTION('center_axis',(1.,0.,0.)) ;
#36600=DIRECTION('ref_axis',(0.,0.,-1.)) ;
#36601=DIRECTION('center_axis',(1.,0.,0.)) ;
#36602=DIRECTION('ref_axis',(0.,0.,-1.)) ;
#36603=DIRECTION('center_axis',(0.,-1.,0.)) ;
#36604=DIRECTION('ref_axis',(1.,0.,0.)) ;
#36605=DIRECTION('',(0.,0.,1.)) ;
#36606=DIRECTION('',(1.,0.,0.)) ;
#36607=DIRECTION('center_axis',(0.,-1.,0.)) ;
#36608=DIRECTION('ref_axis',(1.,0.,0.)) ;
#36609=DIRECTION('',(-1.,0.,0.)) ;
#36610=DIRECTION('',(0.,0.,-1.)) ;
#36611=DIRECTION('center_axis',(0.,0.,1.)) ;
#36612=DIRECTION('ref_axis',(0.,-1.,0.)) ;
#36613=DIRECTION('',(0.,1.,0.)) ;
#36614=DIRECTION('center_axis',(-1.,0.,0.)) ;
#36615=DIRECTION('ref_axis',(0.,-1.,0.)) ;
#36616=DIRECTION('center_axis',(0.,0.,1.)) ;
#36617=DIRECTION('ref_axis',(0.,-1.,0.)) ;
#36618=DIRECTION('',(0.,1.,0.)) ;
#36619=DIRECTION('center_axis',(-1.,0.,0.)) ;
#36620=DIRECTION('ref_axis',(0.,-1.,0.)) ;
#36621=DIRECTION('center_axis',(0.,0.,1.)) ;
#36622=DIRECTION('ref_axis',(1.,0.,0.)) ;
#36623=DIRECTION('',(-1.,0.,0.)) ;
#36624=DIRECTION('',(0.,-1.,0.)) ;
#36625=DIRECTION('center_axis',(0.,1.,0.)) ;
#36626=DIRECTION('ref_axis',(0.,0.,1.)) ;
#36627=DIRECTION('',(0.,0.,-1.)) ;
#36628=DIRECTION('center_axis',(-1.,0.,0.)) ;
#36629=DIRECTION('ref_axis',(0.,0.,1.)) ;
#36630=DIRECTION('center_axis',(1.,0.,0.)) ;
#36631=DIRECTION('ref_axis',(0.,0.,-1.)) ;
#36632=DIRECTION('center_axis',(1.,0.,0.)) ;
#36633=DIRECTION('ref_axis',(0.,0.,-1.)) ;
#36634=DIRECTION('',(-1.,0.,0.)) ;
#36635=DIRECTION('center_axis',(-1.,0.,0.)) ;
#36636=DIRECTION('ref_axis',(0.,0.,-1.)) ;
#36637=DIRECTION('center_axis',(1.,0.,0.)) ;
#36638=DIRECTION('ref_axis',(0.,0.,-1.)) ;
#36639=DIRECTION('center_axis',(-1.,0.,0.)) ;
#36640=DIRECTION('ref_axis',(0.,0.,1.)) ;
#36641=DIRECTION('center_axis',(-1.,0.,0.)) ;
#36642=DIRECTION('ref_axis',(0.,0.,-1.)) ;
#36643=DIRECTION('center_axis',(1.,0.,0.)) ;
#36644=DIRECTION('ref_axis',(0.,0.,-1.)) ;
#36645=DIRECTION('center_axis',(1.,0.,0.)) ;
#36646=DIRECTION('ref_axis',(0.,0.,-1.)) ;
#36647=DIRECTION('',(-1.,0.,0.)) ;
#36648=DIRECTION('center_axis',(1.,0.,0.)) ;
#36649=DIRECTION('ref_axis',(0.,0.,-1.)) ;
#45457=CARTESIAN_POINT('',(0.,0.,0.)) ;
#45458=CARTESIAN_POINT('Origin',(-47.2,0.,34.)) ;
#45459=CARTESIAN_POINT('',(-47.2,-1.72409396495667,33.7)) ;
#45460=CARTESIAN_POINT('',(-47.2,-1.52069063257456,33.7)) ;
#45461=CARTESIAN_POINT('',(-47.2,-0.875,33.7)) ;
#45462=CARTESIAN_POINT('',(-47.2,-1.175,32.7031287650657)) ;
#45463=CARTESIAN_POINT('Origin',(-47.2,0.,34.)) ;
#45464=CARTESIAN_POINT('',(-47.2,-1.175,32.7844555433772)) ;
#45465=CARTESIAN_POINT('',(-47.2,-1.175,33.2422277716886)) ;
#45466=CARTESIAN_POINT('',(-47.2,-0.961744079250633,32.7844555433772)) ;
#45467=CARTESIAN_POINT('',(-47.2,-0.4375,32.7844555433772)) ;
#45468=CARTESIAN_POINT('Origin',(-47.2,0.,34.)) ;
#45469=CARTESIAN_POINT('Origin',(-47.2,0.,34.)) ;
#45470=CARTESIAN_POINT('',(-47.2,-1.52069063257456,34.3)) ;
#45471=CARTESIAN_POINT('',(-47.2,-1.72409396495667,34.3)) ;
#45472=CARTESIAN_POINT('',(-47.2,-0.875,34.3)) ;
#45473=CARTESIAN_POINT('',(-47.2,-0.961744079250633,35.2155444566228)) ;
#45474=CARTESIAN_POINT('Origin',(-47.2,0.,34.)) ;
#45475=CARTESIAN_POINT('',(-47.2,-1.175,35.2155444566228)) ;
#45476=CARTESIAN_POINT('',(-47.2,-0.4375,35.2155444566228)) ;
#45477=CARTESIAN_POINT('',(-47.2,-1.175,35.2968712349343)) ;
#45478=CARTESIAN_POINT('',(-47.2,-1.175,34.7577722283114)) ;
#45479=CARTESIAN_POINT('Origin',(-47.2,0.,34.)) ;
#45480=CARTESIAN_POINT('Origin',(-47.2,0.,34.)) ;
#45481=CARTESIAN_POINT('',(-47.2,-0.575,35.4394009170485)) ;
#45482=CARTESIAN_POINT('',(-47.2,-0.575,35.6528384676066)) ;
#45483=CARTESIAN_POINT('',(-47.2,-0.575,34.7577722283114)) ;
#45484=CARTESIAN_POINT('',(-47.2,0.575,35.4394009170485)) ;
#45485=CARTESIAN_POINT('Origin',(-47.2,0.,34.)) ;
#45486=CARTESIAN_POINT('',(-47.2,0.575,35.6528384676066)) ;
#45487=CARTESIAN_POINT('',(-47.2,0.575,34.7577722283114)) ;
#45488=CARTESIAN_POINT('Origin',(-47.2,0.,34.)) ;
#45489=CARTESIAN_POINT('Origin',(-47.2,0.,34.)) ;
#45490=CARTESIAN_POINT('',(-47.2,0.961744079250633,35.2155444566228)) ;
#45491=CARTESIAN_POINT('',(-47.2,1.175,35.2155444566228)) ;
#45492=CARTESIAN_POINT('',(-47.2,0.4375,35.2155444566228)) ;
#45493=CARTESIAN_POINT('',(-47.2,1.52069063257456,34.3)) ;
#45494=CARTESIAN_POINT('Origin',(-47.2,0.,34.)) ;
#45495=CARTESIAN_POINT('',(-47.2,1.72409396495667,34.3)) ;
#45496=CARTESIAN_POINT('',(-47.2,0.875,34.3)) ;
#45497=CARTESIAN_POINT('',(-47.2,1.175,35.2968712349343)) ;
#45498=CARTESIAN_POINT('Origin',(-47.2,0.,34.)) ;
#45499=CARTESIAN_POINT('',(-47.2,1.175,34.7577722283114)) ;
#45500=CARTESIAN_POINT('Origin',(-47.2,0.,34.)) ;
#45501=CARTESIAN_POINT('',(-47.2,1.52069063257456,33.7)) ;
#45502=CARTESIAN_POINT('',(-47.2,1.72409396495667,33.7)) ;
#45503=CARTESIAN_POINT('',(-47.2,0.875,33.7)) ;
#45504=CARTESIAN_POINT('',(-47.2,0.961744079250633,32.7844555433772)) ;
#45505=CARTESIAN_POINT('Origin',(-47.2,0.,34.)) ;
#45506=CARTESIAN_POINT('',(-47.2,1.175,32.7844555433772)) ;
#45507=CARTESIAN_POINT('',(-47.2,0.4375,32.7844555433772)) ;
#45508=CARTESIAN_POINT('',(-47.2,1.175,32.7031287650657)) ;
#45509=CARTESIAN_POINT('',(-47.2,1.175,33.2422277716886)) ;
#45510=CARTESIAN_POINT('Origin',(-47.2,0.,34.)) ;
#45511=CARTESIAN_POINT('Origin',(-47.2,0.,34.)) ;
#45512=CARTESIAN_POINT('',(-47.2,0.575,32.5605990829515)) ;
#45513=CARTESIAN_POINT('',(-47.2,0.575,32.3471615323934)) ;
#45514=CARTESIAN_POINT('',(-47.2,0.575,33.2422277716886)) ;
#45515=CARTESIAN_POINT('',(-47.2,-0.575000000000001,32.5605990829515)) ;
#45516=CARTESIAN_POINT('Origin',(-47.2,0.,34.)) ;
#45517=CARTESIAN_POINT('',(-47.2,-0.575000000000001,32.3471615323934)) ;
#45518=CARTESIAN_POINT('',(-47.2,-0.575000000000001,33.2422277716886)) ;
#45519=CARTESIAN_POINT('Origin',(-47.2,0.,34.)) ;
#45520=CARTESIAN_POINT('Origin',(-46.9,0.,34.)) ;
#45521=CARTESIAN_POINT('',(-46.6,0.961744079250633,35.2155444566228)) ;
#45522=CARTESIAN_POINT('',(-46.9,0.961744079250633,35.2155444566228)) ;
#45523=CARTESIAN_POINT('',(-46.6,1.52069063257456,34.3)) ;
#45524=CARTESIAN_POINT('Origin',(-46.6,0.,34.)) ;
#45525=CARTESIAN_POINT('',(-46.9,1.52069063257456,34.3)) ;
#45526=CARTESIAN_POINT('Origin',(-46.9,0.,34.)) ;
#45527=CARTESIAN_POINT('',(-46.6,-0.575,35.4394009170485)) ;
#45528=CARTESIAN_POINT('',(-46.9,-0.575,35.4394009170485)) ;
#45529=CARTESIAN_POINT('',(-46.6,0.575,35.4394009170485)) ;
#45530=CARTESIAN_POINT('Origin',(-46.6,0.,34.)) ;
#45531=CARTESIAN_POINT('',(-46.9,0.575,35.4394009170485)) ;
#45532=CARTESIAN_POINT('Origin',(-46.9,0.,34.)) ;
#45533=CARTESIAN_POINT('',(-46.6,-1.52069063257456,33.7)) ;
#45534=CARTESIAN_POINT('',(-46.9,-1.52069063257456,33.7)) ;
#45535=CARTESIAN_POINT('',(-46.6,-0.961744079250633,32.7844555433772)) ;
#45536=CARTESIAN_POINT('',(-46.9,-0.961744079250633,32.7844555433772)) ;
#45537=CARTESIAN_POINT('Origin',(-46.6,0.,34.)) ;
#45538=CARTESIAN_POINT('Origin',(-46.9,0.,34.)) ;
#45539=CARTESIAN_POINT('',(-46.6,-1.52069063257456,34.3)) ;
#45540=CARTESIAN_POINT('',(-46.9,-1.52069063257456,34.3)) ;
#45541=CARTESIAN_POINT('',(-46.6,-0.961744079250633,35.2155444566228)) ;
#45542=CARTESIAN_POINT('Origin',(-46.6,0.,34.)) ;
#45543=CARTESIAN_POINT('',(-46.9,-0.961744079250633,35.2155444566228)) ;
#45544=CARTESIAN_POINT('Origin',(-46.9,0.,34.)) ;
#45545=CARTESIAN_POINT('',(-46.6,1.52069063257456,33.7)) ;
#45546=CARTESIAN_POINT('',(-46.9,1.52069063257456,33.7)) ;
#45547=CARTESIAN_POINT('',(-46.6,0.961744079250633,32.7844555433772)) ;
#45548=CARTESIAN_POINT('Origin',(-46.6,0.,34.)) ;
#45549=CARTESIAN_POINT('',(-46.9,0.961744079250633,32.7844555433772)) ;
#45550=CARTESIAN_POINT('Origin',(-46.9,0.,34.)) ;
#45551=CARTESIAN_POINT('',(-46.6,0.575,32.5605990829515)) ;
#45552=CARTESIAN_POINT('',(-46.9,0.575,32.5605990829515)) ;
#45553=CARTESIAN_POINT('',(-46.6,-0.575000000000001,32.5605990829515)) ;
#45554=CARTESIAN_POINT('Origin',(-46.6,0.,34.)) ;
#45555=CARTESIAN_POINT('',(-46.9,-0.575000000000001,32.5605990829515)) ;
#45556=CARTESIAN_POINT('Origin',(-46.6,0.,34.)) ;
#45557=CARTESIAN_POINT('',(-46.6,-1.72409396495667,33.7)) ;
#45558=CARTESIAN_POINT('',(-46.6,-0.875,33.7)) ;
#45559=CARTESIAN_POINT('',(-46.6,-1.175,32.7844555433772)) ;
#45560=CARTESIAN_POINT('',(-46.6,-0.4375,32.7844555433772)) ;
#45561=CARTESIAN_POINT('',(-46.6,-1.175,32.7031287650657)) ;
#45562=CARTESIAN_POINT('',(-46.6,-1.175,33.2422277716886)) ;
#45563=CARTESIAN_POINT('Origin',(-46.6,0.,34.)) ;
#45564=CARTESIAN_POINT('Origin',(-46.6,0.,34.)) ;
#45565=CARTESIAN_POINT('',(-46.6,-0.575,35.6528384676066)) ;
#45566=CARTESIAN_POINT('',(-46.6,-0.575,34.7577722283114)) ;
#45567=CARTESIAN_POINT('',(-46.6,-2.14313189850787E-16,35.75)) ;
#45568=CARTESIAN_POINT('Origin',(-46.6,0.,34.)) ;
#45569=CARTESIAN_POINT('',(-46.6,0.575,35.6528384676066)) ;
#45570=CARTESIAN_POINT('Origin',(-46.6,0.,34.)) ;
#45571=CARTESIAN_POINT('',(-46.6,0.575,34.7577722283114)) ;
#45572=CARTESIAN_POINT('Origin',(-46.6,0.,34.)) ;
#45573=CARTESIAN_POINT('',(-46.6,1.175,35.2155444566228)) ;
#45574=CARTESIAN_POINT('',(-46.6,0.4375,35.2155444566228)) ;
#45575=CARTESIAN_POINT('',(-46.6,1.175,35.2968712349343)) ;
#45576=CARTESIAN_POINT('',(-46.6,1.175,34.7577722283114)) ;
#45577=CARTESIAN_POINT('',(-46.6,1.72409396495667,34.3)) ;
#45578=CARTESIAN_POINT('Origin',(-46.6,0.,34.)) ;
#45579=CARTESIAN_POINT('',(-46.6,0.875,34.3)) ;
#45580=CARTESIAN_POINT('Origin',(-46.6,0.,34.)) ;
#45581=CARTESIAN_POINT('',(-46.6,1.72409396495667,33.7)) ;
#45582=CARTESIAN_POINT('',(-46.6,0.875,33.7)) ;
#45583=CARTESIAN_POINT('',(-46.6,1.175,32.7031287650657)) ;
#45584=CARTESIAN_POINT('Origin',(-46.6,0.,34.)) ;
#45585=CARTESIAN_POINT('',(-46.6,1.175,32.7844555433772)) ;
#45586=CARTESIAN_POINT('',(-46.6,1.175,33.2422277716886)) ;
#45587=CARTESIAN_POINT('',(-46.6,0.4375,32.7844555433772)) ;
#45588=CARTESIAN_POINT('Origin',(-46.6,0.,34.)) ;
#45589=CARTESIAN_POINT('',(-46.6,-1.72409396495667,34.3)) ;
#45590=CARTESIAN_POINT('',(-46.6,-0.875,34.3)) ;
#45591=CARTESIAN_POINT('',(-46.6,-1.175,35.2968712349343)) ;
#45592=CARTESIAN_POINT('Origin',(-46.6,0.,34.)) ;
#45593=CARTESIAN_POINT('',(-46.6,-1.175,35.2155444566228)) ;
#45594=CARTESIAN_POINT('',(-46.6,-1.175,34.7577722283114)) ;
#45595=CARTESIAN_POINT('',(-46.6,-0.4375,35.2155444566228)) ;
#45596=CARTESIAN_POINT('Origin',(-46.6,0.,34.)) ;
#45597=CARTESIAN_POINT('',(-46.6,0.575,32.3471615323934)) ;
#45598=CARTESIAN_POINT('',(-46.6,0.575,33.2422277716886)) ;
#45599=CARTESIAN_POINT('',(-46.6,-0.575000000000001,32.3471615323934)) ;
#45600=CARTESIAN_POINT('Origin',(-46.6,0.,34.)) ;
#45601=CARTESIAN_POINT('',(-46.6,-0.575000000000001,33.2422277716886)) ;
#45602=CARTESIAN_POINT('Origin',(-48.,0.575,32.4844555433772)) ;
#45603=CARTESIAN_POINT('',(-52.,0.575,32.3471615323934)) ;
#45604=CARTESIAN_POINT('',(-45.,0.575,32.3471615323934)) ;
#45605=CARTESIAN_POINT('',(-52.,0.575,32.7844555433772)) ;
#45606=CARTESIAN_POINT('',(-52.,0.575,33.2422277716886)) ;
#45607=CARTESIAN_POINT('',(-44.,0.575,32.7844555433772)) ;
#45608=CARTESIAN_POINT('',(-48.,0.575,32.7844555433772)) ;
#45609=CARTESIAN_POINT('',(-44.,0.575,32.3471615323934)) ;
#45610=CARTESIAN_POINT('',(-44.,0.575,32.4844555433772)) ;
#45611=CARTESIAN_POINT('',(-45.,0.575,32.3471615323934)) ;
#45612=CARTESIAN_POINT('Origin',(-48.,-1.75,34.3)) ;
#45613=CARTESIAN_POINT('',(-52.,-1.72409396495667,34.3)) ;
#45614=CARTESIAN_POINT('',(-45.,-1.72409396495667,34.3)) ;
#45615=CARTESIAN_POINT('',(-52.,-1.45,34.3)) ;
#45616=CARTESIAN_POINT('',(-52.,-0.875,34.3)) ;
#45617=CARTESIAN_POINT('',(-44.,-1.45,34.3)) ;
#45618=CARTESIAN_POINT('',(-48.,-1.45,34.3)) ;
#45619=CARTESIAN_POINT('',(-44.,-1.72409396495667,34.3)) ;
#45620=CARTESIAN_POINT('',(-44.,-1.75,34.3)) ;
#45621=CARTESIAN_POINT('',(-45.,-1.72409396495667,34.3)) ;
#45622=CARTESIAN_POINT('Origin',(-48.,-1.175,35.5155444566228)) ;
#45623=CARTESIAN_POINT('',(-52.,-1.175,35.2155444566228)) ;
#45624=CARTESIAN_POINT('',(-48.,-1.175,35.2155444566228)) ;
#45625=CARTESIAN_POINT('',(-52.,-1.175,35.2968712349343)) ;
#45626=CARTESIAN_POINT('',(-52.,-1.175,34.7577722283114)) ;
#45627=CARTESIAN_POINT('',(-45.,-1.175,35.2968712349343)) ;
#45628=CARTESIAN_POINT('Origin',(-48.,0.875,32.7844555433772)) ;
#45629=CARTESIAN_POINT('',(-44.,1.175,32.7844555433772)) ;
#45630=CARTESIAN_POINT('',(-48.,1.175,32.7844555433772)) ;
#45631=CARTESIAN_POINT('',(-44.,0.875,32.7844555433772)) ;
#45632=CARTESIAN_POINT('',(-52.,1.175,32.7844555433772)) ;
#45633=CARTESIAN_POINT('',(-52.,0.4375,32.7844555433772)) ;
#45634=CARTESIAN_POINT('',(-48.,1.175,32.7844555433772)) ;
#45635=CARTESIAN_POINT('Origin',(-48.,1.175,32.4844555433772)) ;
#45636=CARTESIAN_POINT('',(-44.,1.175,32.7031287650657)) ;
#45637=CARTESIAN_POINT('',(-45.,1.175,32.7031287650657)) ;
#45638=CARTESIAN_POINT('',(-44.,1.175,32.4844555433772)) ;
#45639=CARTESIAN_POINT('Origin',(-48.,1.175,32.4844555433772)) ;
#45640=CARTESIAN_POINT('',(-52.,1.175,32.7031287650657)) ;
#45641=CARTESIAN_POINT('',(-52.,1.175,33.2422277716886)) ;
#45642=CARTESIAN_POINT('',(-45.,1.175,32.7031287650657)) ;
#45643=CARTESIAN_POINT('Origin',(-48.,-1.75,33.7)) ;
#45644=CARTESIAN_POINT('',(-44.,-1.72409396495667,33.7)) ;
#45645=CARTESIAN_POINT('',(-45.,-1.72409396495667,33.7)) ;
#45646=CARTESIAN_POINT('',(-44.,-1.45,33.7)) ;
#45647=CARTESIAN_POINT('',(-44.,-1.75,33.7)) ;
#45648=CARTESIAN_POINT('',(-52.,-1.45,33.7)) ;
#45649=CARTESIAN_POINT('',(-48.,-1.45,33.7)) ;
#45650=CARTESIAN_POINT('',(-52.,-1.72409396495667,33.7)) ;
#45651=CARTESIAN_POINT('',(-52.,-0.875,33.7)) ;
#45652=CARTESIAN_POINT('',(-45.,-1.72409396495667,33.7)) ;
#45653=CARTESIAN_POINT('Origin',(-48.,-1.175,32.4844555433772)) ;
#45654=CARTESIAN_POINT('',(-44.,-1.175,32.7844555433772)) ;
#45655=CARTESIAN_POINT('',(-48.,-1.175,32.7844555433772)) ;
#45656=CARTESIAN_POINT('',(-44.,-1.175,32.7031287650657)) ;
#45657=CARTESIAN_POINT('',(-44.,-1.175,32.4844555433772)) ;
#45658=CARTESIAN_POINT('',(-45.,-1.175,32.7031287650657)) ;
#45659=CARTESIAN_POINT('Origin',(-48.,1.75,34.3)) ;
#45660=CARTESIAN_POINT('',(-44.,1.72409396495667,34.3)) ;
#45661=CARTESIAN_POINT('',(-45.,1.72409396495667,34.3)) ;
#45662=CARTESIAN_POINT('',(-44.,1.45,34.3)) ;
#45663=CARTESIAN_POINT('',(-44.,1.75,34.3)) ;
#45664=CARTESIAN_POINT('',(-52.,1.45,34.3)) ;
#45665=CARTESIAN_POINT('',(-48.,1.45,34.3)) ;
#45666=CARTESIAN_POINT('',(-52.,1.72409396495667,34.3)) ;
#45667=CARTESIAN_POINT('',(-52.,0.875,34.3)) ;
#45668=CARTESIAN_POINT('',(-45.,1.72409396495667,34.3)) ;
#45669=CARTESIAN_POINT('Origin',(-48.,1.175,35.5155444566228)) ;
#45670=CARTESIAN_POINT('',(-44.,1.175,35.2155444566228)) ;
#45671=CARTESIAN_POINT('',(-48.,1.175,35.2155444566228)) ;
#45672=CARTESIAN_POINT('',(-44.,1.175,35.2968712349343)) ;
#45673=CARTESIAN_POINT('',(-44.,1.175,35.5155444566228)) ;
#45674=CARTESIAN_POINT('',(-45.,1.175,35.2968712349343)) ;
#45675=CARTESIAN_POINT('Origin',(-48.,1.175,35.5155444566228)) ;
#45676=CARTESIAN_POINT('',(-52.,1.175,35.2968712349343)) ;
#45677=CARTESIAN_POINT('',(-45.,1.175,35.2968712349343)) ;
#45678=CARTESIAN_POINT('',(-52.,1.175,35.2155444566228)) ;
#45679=CARTESIAN_POINT('',(-52.,1.175,34.7577722283114)) ;
#45680=CARTESIAN_POINT('',(-48.,1.175,35.2155444566228)) ;
#45681=CARTESIAN_POINT('Origin',(-48.,0.575,35.5155444566228)) ;
#45682=CARTESIAN_POINT('',(-44.,0.575,35.6528384676066)) ;
#45683=CARTESIAN_POINT('',(-45.,0.575,35.6528384676066)) ;
#45684=CARTESIAN_POINT('',(-44.,0.575,35.2155444566228)) ;
#45685=CARTESIAN_POINT('',(-44.,0.575,35.5155444566228)) ;
#45686=CARTESIAN_POINT('',(-52.,0.575,35.2155444566228)) ;
#45687=CARTESIAN_POINT('',(-48.,0.575,35.2155444566228)) ;
#45688=CARTESIAN_POINT('',(-52.,0.575,35.6528384676066)) ;
#45689=CARTESIAN_POINT('',(-52.,0.575,34.7577722283114)) ;
#45690=CARTESIAN_POINT('',(-45.,0.575,35.6528384676066)) ;
#45691=CARTESIAN_POINT('Origin',(-45.,0.,34.)) ;
#45692=CARTESIAN_POINT('',(-52.,-0.575,35.6528384676066)) ;
#45693=CARTESIAN_POINT('Origin',(-52.,0.,34.)) ;
#45694=CARTESIAN_POINT('',(-45.,-0.575,35.6528384676066)) ;
#45695=CARTESIAN_POINT('Origin',(-45.,0.,34.)) ;
#45696=CARTESIAN_POINT('Origin',(-52.,0.,34.)) ;
#45697=CARTESIAN_POINT('Origin',(-45.,0.,34.)) ;
#45698=CARTESIAN_POINT('',(-52.,1.72409396495667,33.7)) ;
#45699=CARTESIAN_POINT('Origin',(-52.,0.,34.)) ;
#45700=CARTESIAN_POINT('',(-45.,1.72409396495667,33.7)) ;
#45701=CARTESIAN_POINT('Origin',(-45.,0.,34.)) ;
#45702=CARTESIAN_POINT('',(-52.,-1.175,32.7031287650657)) ;
#45703=CARTESIAN_POINT('Origin',(-52.,0.,34.)) ;
#45704=CARTESIAN_POINT('',(-45.,-1.175,32.7031287650657)) ;
#45705=CARTESIAN_POINT('Origin',(-45.,0.,34.)) ;
#45706=CARTESIAN_POINT('Origin',(-52.,0.,34.)) ;
#45707=CARTESIAN_POINT('Origin',(-45.,0.,34.)) ;
#45708=CARTESIAN_POINT('',(-52.,-0.575000000000001,32.3471615323934)) ;
#45709=CARTESIAN_POINT('',(-45.,-0.575000000000001,32.3471615323934)) ;
#45710=CARTESIAN_POINT('Origin',(-52.,0.,34.)) ;
#45711=CARTESIAN_POINT('Origin',(-44.,0.875,32.4844555433772)) ;
#45712=CARTESIAN_POINT('Origin',(-44.,0.,34.)) ;
#45713=CARTESIAN_POINT('Origin',(-52.,0.,34.)) ;
#45714=CARTESIAN_POINT('',(-52.,-0.575000000000001,32.7844555433772)) ;
#45715=CARTESIAN_POINT('',(-52.,-0.575000000000001,33.2422277716886)) ;
#45716=CARTESIAN_POINT('',(-52.,-1.175,32.7844555433772)) ;
#45717=CARTESIAN_POINT('',(-52.,-0.4375,32.7844555433772)) ;
#45718=CARTESIAN_POINT('',(-52.,-1.175,33.2422277716886)) ;
#45719=CARTESIAN_POINT('',(-52.,-1.45,34.)) ;
#45720=CARTESIAN_POINT('',(-52.,-0.575,35.2155444566228)) ;
#45721=CARTESIAN_POINT('',(-52.,-0.4375,35.2155444566228)) ;
#45722=CARTESIAN_POINT('',(-52.,-0.575,34.7577722283114)) ;
#45723=CARTESIAN_POINT('',(-52.,0.4375,35.2155444566228)) ;
#45724=CARTESIAN_POINT('',(-52.,1.45,33.7)) ;
#45725=CARTESIAN_POINT('',(-52.,1.45,34.)) ;
#45726=CARTESIAN_POINT('',(-52.,0.875,33.7)) ;
#45727=CARTESIAN_POINT('Origin',(-48.,-0.575000000000001,32.4844555433772)) ;
#45728=CARTESIAN_POINT('',(-44.,-0.575000000000001,32.3471615323934)) ;
#45729=CARTESIAN_POINT('',(-45.,-0.575000000000001,32.3471615323934)) ;
#45730=CARTESIAN_POINT('',(-44.,-0.575000000000001,32.7844555433772)) ;
#45731=CARTESIAN_POINT('',(-44.,-0.575000000000001,32.4844555433772)) ;
#45732=CARTESIAN_POINT('',(-48.,-0.575000000000001,32.7844555433772)) ;
#45733=CARTESIAN_POINT('Origin',(-48.,-1.175,32.4844555433772)) ;
#45734=CARTESIAN_POINT('',(-48.,-1.175,32.7844555433772)) ;
#45735=CARTESIAN_POINT('Origin',(-48.,-0.875000000000001,32.7844555433772)) ;
#45736=CARTESIAN_POINT('',(-44.,-0.875000000000001,32.7844555433772)) ;
#45737=CARTESIAN_POINT('Origin',(-44.,-0.875000000000001,32.4844555433772)) ;
#45738=CARTESIAN_POINT('Origin',(-44.,0.,34.)) ;
#45739=CARTESIAN_POINT('Origin',(-44.,-1.75,34.)) ;
#45740=CARTESIAN_POINT('Origin',(-44.,0.,34.)) ;
#45741=CARTESIAN_POINT('',(-44.,-1.45,34.)) ;
#45742=CARTESIAN_POINT('Origin',(-48.,-1.45,34.)) ;
#45743=CARTESIAN_POINT('Origin',(-45.,0.,34.)) ;
#45744=CARTESIAN_POINT('',(-38.,-2.14313189850787E-16,35.75)) ;
#45745=CARTESIAN_POINT('Origin',(-38.,0.,34.)) ;
#45746=CARTESIAN_POINT('',(-45.,-2.14313189850787E-16,35.75)) ;
#45747=CARTESIAN_POINT('',(-44.,-0.575,35.6528384676066)) ;
#45748=CARTESIAN_POINT('',(-45.,-0.575,35.6528384676066)) ;
#45749=CARTESIAN_POINT('',(-44.,-1.175,35.2968712349343)) ;
#45750=CARTESIAN_POINT('Origin',(-44.,0.,34.)) ;
#45751=CARTESIAN_POINT('',(-45.,-1.175,35.2968712349343)) ;
#45752=CARTESIAN_POINT('',(-44.,1.72409396495667,33.7)) ;
#45753=CARTESIAN_POINT('',(-45.,1.72409396495667,33.7)) ;
#45754=CARTESIAN_POINT('Origin',(-44.,0.,34.)) ;
#45755=CARTESIAN_POINT('Origin',(-44.,0.,34.)) ;
#45756=CARTESIAN_POINT('Origin',(-48.,-1.175,35.5155444566228)) ;
#45757=CARTESIAN_POINT('',(-44.,-1.175,35.2155444566228)) ;
#45758=CARTESIAN_POINT('',(-44.,-1.175,35.5155444566228)) ;
#45759=CARTESIAN_POINT('',(-48.,-1.175,35.2155444566228)) ;
#45760=CARTESIAN_POINT('Origin',(-48.,-0.575,35.5155444566228)) ;
#45761=CARTESIAN_POINT('',(-44.,-0.575,35.2155444566228)) ;
#45762=CARTESIAN_POINT('',(-48.,-0.575,35.2155444566228)) ;
#45763=CARTESIAN_POINT('',(-44.,-0.575,35.5155444566228)) ;
#45764=CARTESIAN_POINT('Origin',(-48.,-0.875,35.2155444566228)) ;
#45765=CARTESIAN_POINT('',(-44.,-0.875,35.2155444566228)) ;
#45766=CARTESIAN_POINT('Origin',(-44.,-0.875,35.5155444566228)) ;
#45767=CARTESIAN_POINT('Origin',(-48.,0.875,35.2155444566228)) ;
#45768=CARTESIAN_POINT('',(-44.,0.875,35.2155444566228)) ;
#45769=CARTESIAN_POINT('Origin',(-44.,0.875,35.5155444566228)) ;
#45770=CARTESIAN_POINT('Origin',(-48.,1.75,33.7)) ;
#45771=CARTESIAN_POINT('',(-44.,1.45,33.7)) ;
#45772=CARTESIAN_POINT('',(-48.,1.45,33.7)) ;
#45773=CARTESIAN_POINT('',(-44.,1.75,33.7)) ;
#45774=CARTESIAN_POINT('Origin',(-48.,1.45,34.)) ;
#45775=CARTESIAN_POINT('',(-44.,1.45,34.)) ;
#45776=CARTESIAN_POINT('Origin',(-44.,1.75,34.)) ;
#45777=CARTESIAN_POINT('Origin',(-33.5,0.,34.)) ;
#45778=CARTESIAN_POINT('',(-30.,-2.14313189850787E-16,35.75)) ;
#45779=CARTESIAN_POINT('Origin',(-30.,0.,34.)) ;
#45780=CARTESIAN_POINT('',(-37.,-2.14313189850787E-16,35.75)) ;
#45781=CARTESIAN_POINT('',(-33.5,-2.14313189850787E-16,35.75)) ;
#45782=CARTESIAN_POINT('Origin',(-37.,0.,34.)) ;
#45783=CARTESIAN_POINT('Origin',(-30.,0.,34.)) ;
#45784=CARTESIAN_POINT('Origin',(-38.,0.,34.)) ;
#45785=CARTESIAN_POINT('',(-38.,-2.69422295812418E-16,36.2)) ;
#45786=CARTESIAN_POINT('Origin',(-38.,0.,34.)) ;
#45787=CARTESIAN_POINT('Origin',(-37.5,0.,34.)) ;
#45788=CARTESIAN_POINT('',(-37.,-2.69422295812418E-16,36.2)) ;
#45789=CARTESIAN_POINT('Origin',(-37.,0.,34.)) ;
#45790=CARTESIAN_POINT('',(-37.5,-2.69422295812418E-16,36.2)) ;
#45791=CARTESIAN_POINT('Origin',(-37.,0.,34.)) ;
#50350=UNCERTAINTY_MEASURE_WITH_UNIT(LENGTH_MEASURE(0.001),#50441,
'DISTANCE_ACCURACY_VALUE',
'Maximum model space distance between geometric entities at asserted c
onnectivities') ;
#50387=UNCERTAINTY_MEASURE_WITH_UNIT(LENGTH_MEASURE(0.001),#50441,
'DISTANCE_ACCURACY_VALUE',
'Maximum model space distance between geometric entities at asserted c
onnectivities') ;
#50403=(
GEOMETRIC_REPRESENTATION_CONTEXT(3)
GLOBAL_UNCERTAINTY_ASSIGNED_CONTEXT((#50350))
GLOBAL_UNIT_ASSIGNED_CONTEXT((#50441,#50443,#50444))
REPRESENTATION_CONTEXT('','3D')
) ;
#50440=(
GEOMETRIC_REPRESENTATION_CONTEXT(3)
GLOBAL_UNCERTAINTY_ASSIGNED_CONTEXT((#50387))
GLOBAL_UNIT_ASSIGNED_CONTEXT((#50441,#50443,#50444))
REPRESENTATION_CONTEXT('','3D')
) ;
#50441=(
LENGTH_UNIT()
NAMED_UNIT(*)
SI_UNIT(.CENTI.,.METRE.)
) ;
#50443=(
NAMED_UNIT(*)
PLANE_ANGLE_UNIT()
SI_UNIT($,.RADIAN.)
) ;
#50444=(
NAMED_UNIT(*)
SI_UNIT($,.STERADIAN.)
SOLID_ANGLE_UNIT()
) ;
#50460=SHAPE_DEFINITION_REPRESENTATION(#50526,#50634) ;
#50526=PRODUCT_DEFINITION_SHAPE('',$,#50687) ;
#50634=SHAPE_REPRESENTATION('',(#30407),#50403) ;
#50671=PRODUCT_DEFINITION_CONTEXT('part definition',#50829,'design') ;
#50687=PRODUCT_DEFINITION('PTO_INPUT_SHAFT_SPLINE',
'PTO_INPUT_SHAFT_SPLINE',#50739,#50671) ;
#50739=PRODUCT_DEFINITION_FORMATION('',$,#50846) ;
#50829=APPLICATION_CONTEXT(
'Core Data for Automotive Mechanical Design Process') ;
#50830=PRODUCT_CONTEXT('part definition',#50829,'mechanical') ;
#50846=PRODUCT('PTO_INPUT_SHAFT_SPLINE','PTO_INPUT_SHAFT_SPLINE',$,(#50830)) ;
#50883=PRESENTATION_STYLE_ASSIGNMENT((#50890)) ;
#50890=SURFACE_STYLE_USAGE(.BOTH.,#50897) ;
#50897=SURFACE_SIDE_STYLE('',(#50904)) ;
#50904=SURFACE_STYLE_FILL_AREA(#50911) ;
#50911=FILL_AREA_STYLE('Steel - Satin',(#50918)) ;
#50918=FILL_AREA_STYLE_COLOUR('Steel - Satin',#50925) ;
#50925=COLOUR_RGB('Steel - Satin', 0.31764706, 0.68627451, 0.89019608) ;
ENDSEC;
END-ISO-10303-21;
